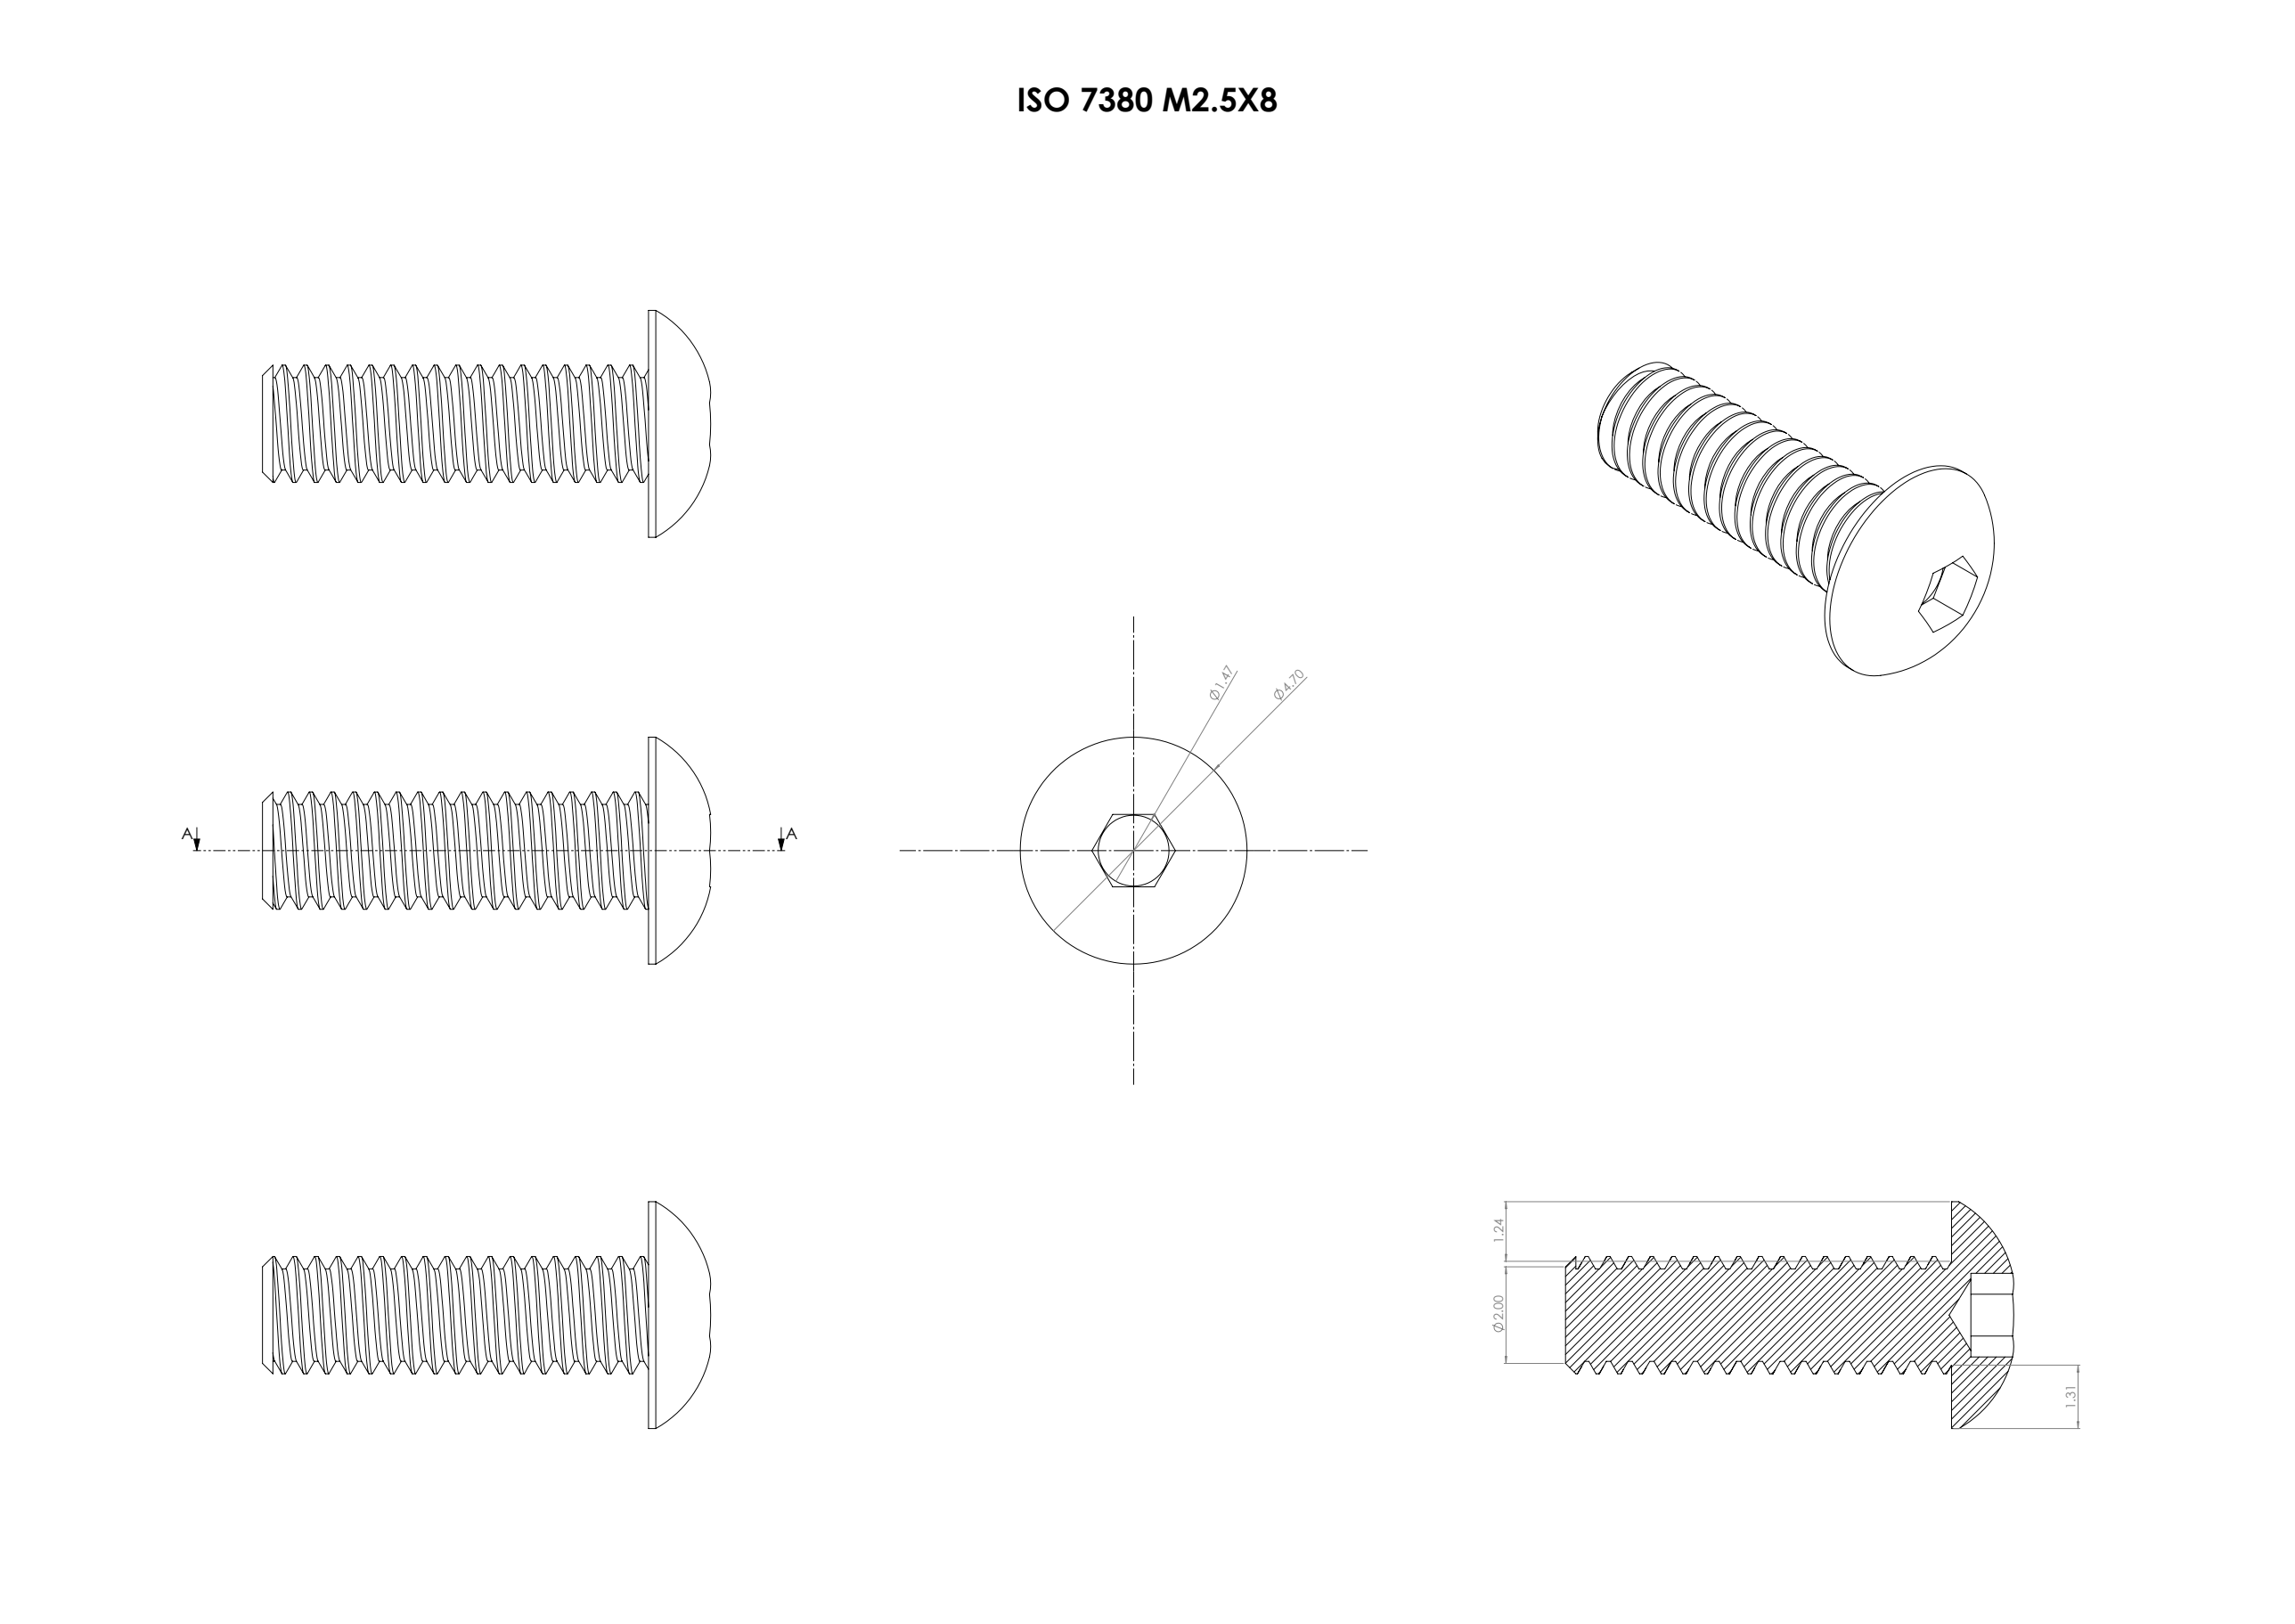
ISO-10303-21;
HEADER;
/* Generated by software containing ST-Developer
 * from STEP Tools, Inc. (www.steptools.com) 
 */

FILE_DESCRIPTION(
/* description */ (''),
/* implementation_level */ '2;1');

FILE_NAME(
/* name */ '13_ISO_7380_M2.5x8.step',
/* time_stamp */ '2026-10-21T02:01:14-07:00',
/* author */ (''),
/* organization */ (''),
/* preprocessor_version */ 'ST-DEVELOPER v20.2',
/* originating_system */ 'Autodesk Translation Framework v15.15.0.0',
/* authorisation */ '');

FILE_SCHEMA (('AUTOMOTIVE_DESIGN { 1 0 10303 214 3 1 1 }'));
ENDSEC;

DATA;
#10=MECHANICAL_DESIGN_GEOMETRIC_PRESENTATION_REPRESENTATION('',(#626),#37181);
#104=(
BOUNDED_SURFACE()
B_SPLINE_SURFACE(2,2,((#37099,#37100,#37101,#37102,#37103,#37104,#37105,
#37106,#37107),(#37108,#37109,#37110,#37111,#37112,#37113,#37114,#37115,
#37116),(#37117,#37118,#37119,#37120,#37121,#37122,#37123,#37124,#37125)),
 .UNSPECIFIED.,.F.,.T.,.F.)
B_SPLINE_SURFACE_WITH_KNOTS((3,3),(3,2,2,2,3),(0.513408172091738,1.39168804086818),
(-3.14159265358979,-1.5707963267949,0.,1.5707963267949,3.14159265358979),
 .UNSPECIFIED.)
GEOMETRIC_REPRESENTATION_ITEM()
RATIONAL_B_SPLINE_SURFACE(((1.,0.707106781186548,1.,0.707106781186548,1.,
0.707106781186548,1.,0.707106781186548,1.),(0.905117664433204,0.640014838292448,
0.905117664433204,0.640014838292448,0.905117664433204,0.640014838292448,
0.905117664433204,0.640014838292448,0.905117664433204),(1.,0.707106781186548,
1.,0.707106781186548,1.,0.707106781186548,1.,0.707106781186548,1.)))
REPRESENTATION_ITEM('')
SURFACE()
);
#118=B_SPLINE_SURFACE_WITH_KNOTS('',3,3,((#35741,#35742,#35743,#35744,#35745,
#35746,#35747,#35748,#35749,#35750,#35751,#35752,#35753,#35754,#35755,#35756,
#35757,#35758,#35759,#35760,#35761,#35762,#35763,#35764,#35765,#35766,#35767,
#35768,#35769,#35770,#35771,#35772,#35773,#35774,#35775,#35776,#35777,#35778,
#35779,#35780,#35781,#35782,#35783,#35784,#35785,#35786,#35787,#35788,#35789,
#35790,#35791,#35792,#35793,#35794,#35795,#35796,#35797,#35798,#35799,#35800,
#35801,#35802,#35803,#35804,#35805,#35806,#35807,#35808,#35809,#35810,#35811,
#35812,#35813,#35814,#35815,#35816,#35817,#35818,#35819,#35820,#35821,#35822,
#35823,#35824,#35825,#35826,#35827,#35828,#35829,#35830,#35831,#35832,#35833,
#35834,#35835,#35836,#35837,#35838,#35839,#35840,#35841,#35842,#35843,#35844,
#35845,#35846,#35847,#35848,#35849,#35850,#35851,#35852,#35853,#35854),
(#35855,#35856,#35857,#35858,#35859,#35860,#35861,#35862,#35863,#35864,
#35865,#35866,#35867,#35868,#35869,#35870,#35871,#35872,#35873,#35874,#35875,
#35876,#35877,#35878,#35879,#35880,#35881,#35882,#35883,#35884,#35885,#35886,
#35887,#35888,#35889,#35890,#35891,#35892,#35893,#35894,#35895,#35896,#35897,
#35898,#35899,#35900,#35901,#35902,#35903,#35904,#35905,#35906,#35907,#35908,
#35909,#35910,#35911,#35912,#35913,#35914,#35915,#35916,#35917,#35918,#35919,
#35920,#35921,#35922,#35923,#35924,#35925,#35926,#35927,#35928,#35929,#35930,
#35931,#35932,#35933,#35934,#35935,#35936,#35937,#35938,#35939,#35940,#35941,
#35942,#35943,#35944,#35945,#35946,#35947,#35948,#35949,#35950,#35951,#35952,
#35953,#35954,#35955,#35956,#35957,#35958,#35959,#35960,#35961,#35962,#35963,
#35964,#35965,#35966,#35967,#35968),(#35969,#35970,#35971,#35972,#35973,
#35974,#35975,#35976,#35977,#35978,#35979,#35980,#35981,#35982,#35983,#35984,
#35985,#35986,#35987,#35988,#35989,#35990,#35991,#35992,#35993,#35994,#35995,
#35996,#35997,#35998,#35999,#36000,#36001,#36002,#36003,#36004,#36005,#36006,
#36007,#36008,#36009,#36010,#36011,#36012,#36013,#36014,#36015,#36016,#36017,
#36018,#36019,#36020,#36021,#36022,#36023,#36024,#36025,#36026,#36027,#36028,
#36029,#36030,#36031,#36032,#36033,#36034,#36035,#36036,#36037,#36038,#36039,
#36040,#36041,#36042,#36043,#36044,#36045,#36046,#36047,#36048,#36049,#36050,
#36051,#36052,#36053,#36054,#36055,#36056,#36057,#36058,#36059,#36060,#36061,
#36062,#36063,#36064,#36065,#36066,#36067,#36068,#36069,#36070,#36071,#36072,
#36073,#36074,#36075,#36076,#36077,#36078,#36079,#36080,#36081,#36082),
(#36083,#36084,#36085,#36086,#36087,#36088,#36089,#36090,#36091,#36092,
#36093,#36094,#36095,#36096,#36097,#36098,#36099,#36100,#36101,#36102,#36103,
#36104,#36105,#36106,#36107,#36108,#36109,#36110,#36111,#36112,#36113,#36114,
#36115,#36116,#36117,#36118,#36119,#36120,#36121,#36122,#36123,#36124,#36125,
#36126,#36127,#36128,#36129,#36130,#36131,#36132,#36133,#36134,#36135,#36136,
#36137,#36138,#36139,#36140,#36141,#36142,#36143,#36144,#36145,#36146,#36147,
#36148,#36149,#36150,#36151,#36152,#36153,#36154,#36155,#36156,#36157,#36158,
#36159,#36160,#36161,#36162,#36163,#36164,#36165,#36166,#36167,#36168,#36169,
#36170,#36171,#36172,#36173,#36174,#36175,#36176,#36177,#36178,#36179,#36180,
#36181,#36182,#36183,#36184,#36185,#36186,#36187,#36188,#36189,#36190,#36191,
#36192,#36193,#36194,#36195,#36196)),.UNSPECIFIED.,.F.,.F.,.F.,(4,4),(4,
1,1,1,1,1,1,1,1,1,1,1,1,1,1,1,1,1,1,1,1,1,1,1,1,1,1,1,1,1,1,1,1,1,1,1,1,
1,1,1,1,1,1,1,1,1,1,1,1,1,1,1,1,1,1,1,1,1,1,1,1,1,1,1,1,1,1,1,1,1,1,1,1,
1,1,1,1,1,1,1,1,1,1,1,1,1,1,1,1,1,1,1,1,1,1,1,1,1,1,1,1,1,1,1,1,1,1,1,1,
1,1,4),(0.,0.0296469363228873),(8.30626835282484,9.30418594221277,10.3021035316007,
11.3000211209886,12.2979387103766,13.2958562997645,14.2937738891524,15.2916914785404,
16.2896090679283,17.2875266573163,18.2854442467042,19.2833618360921,20.2812794254801,
21.279197014868,22.2771146042559,23.2750321936439,24.2729497830318,25.2708673724197,
26.2687849618077,27.2667025511956,28.2646201405835,29.2625377299715,30.2604553193594,
31.2583729087473,32.2562904981353,33.2542080875232,34.2521256769111,35.2500432662991,
36.247960855687,37.245878445075,38.2437960344629,39.2417136238508,40.2396312132388,
41.2375488026267,42.2354663920146,43.2333839814026,44.2313015707905,45.2292191601784,
46.2271367495664,47.2250543389543,48.2229719283422,49.2208895177302,50.2188071071181,
51.216724696506,52.214642285894,53.2125598752819,54.2104774646699,55.2083950540578,
56.2063126434457,57.2042302328337,58.2021478222216,59.2000654116095,60.1979830009975,
61.1959005903854,62.1938181797733,63.1917357691613,64.1896533585492,65.1875709479371,
66.1854885373251,67.183406126713,68.1813237161009,69.1792413054889,70.1771588948768,
71.1750764842647,72.1729940736527,73.1709116630406,74.1688292524286,75.1667468418165,
76.1646644312044,77.1625820205924,78.1604996099803,79.1584171993682,80.1563347887562,
81.1542523781441,82.152169967532,83.15008755692,84.1480051463079,85.1459227356958,
86.1438403250838,87.1417579144717,88.1396755038596,89.1375930932476,90.1355106826355,
91.1334282720235,92.1313458614114,93.1292634507993,94.1271810401873,95.1250986295752,
96.1230162189631,97.1209338083511,98.118851397739,99.1167689871269,100.114686576515,
101.112604165903,102.110521755291,103.108439344679,104.106356934067,105.104274523455,
106.102192112842,107.10010970223,108.098027291618,109.095944881006,110.093862470394,
111.091780059782,112.08969764917,113.087615238558,114.085532827946,115.083450417334,
116.081368006722,117.07928559611,118.077203185498,119.075120774886),
 .UNSPECIFIED.);
#119=B_SPLINE_SURFACE_WITH_KNOTS('',3,3,((#36473,#36474,#36475,#36476,#36477,
#36478,#36479,#36480,#36481,#36482,#36483,#36484,#36485,#36486,#36487,#36488,
#36489,#36490,#36491,#36492,#36493,#36494,#36495,#36496,#36497,#36498,#36499,
#36500,#36501,#36502,#36503,#36504,#36505,#36506,#36507,#36508,#36509,#36510,
#36511,#36512,#36513,#36514,#36515,#36516,#36517,#36518,#36519,#36520,#36521,
#36522,#36523,#36524,#36525,#36526,#36527,#36528,#36529,#36530,#36531,#36532,
#36533,#36534,#36535,#36536,#36537,#36538,#36539,#36540,#36541,#36542,#36543,
#36544,#36545,#36546,#36547,#36548,#36549,#36550,#36551,#36552,#36553,#36554,
#36555,#36556,#36557,#36558,#36559,#36560,#36561,#36562,#36563,#36564,#36565,
#36566,#36567,#36568,#36569,#36570,#36571,#36572,#36573,#36574,#36575,#36576,
#36577,#36578,#36579,#36580,#36581,#36582,#36583,#36584,#36585,#36586),
(#36587,#36588,#36589,#36590,#36591,#36592,#36593,#36594,#36595,#36596,
#36597,#36598,#36599,#36600,#36601,#36602,#36603,#36604,#36605,#36606,#36607,
#36608,#36609,#36610,#36611,#36612,#36613,#36614,#36615,#36616,#36617,#36618,
#36619,#36620,#36621,#36622,#36623,#36624,#36625,#36626,#36627,#36628,#36629,
#36630,#36631,#36632,#36633,#36634,#36635,#36636,#36637,#36638,#36639,#36640,
#36641,#36642,#36643,#36644,#36645,#36646,#36647,#36648,#36649,#36650,#36651,
#36652,#36653,#36654,#36655,#36656,#36657,#36658,#36659,#36660,#36661,#36662,
#36663,#36664,#36665,#36666,#36667,#36668,#36669,#36670,#36671,#36672,#36673,
#36674,#36675,#36676,#36677,#36678,#36679,#36680,#36681,#36682,#36683,#36684,
#36685,#36686,#36687,#36688,#36689,#36690,#36691,#36692,#36693,#36694,#36695,
#36696,#36697,#36698,#36699,#36700),(#36701,#36702,#36703,#36704,#36705,
#36706,#36707,#36708,#36709,#36710,#36711,#36712,#36713,#36714,#36715,#36716,
#36717,#36718,#36719,#36720,#36721,#36722,#36723,#36724,#36725,#36726,#36727,
#36728,#36729,#36730,#36731,#36732,#36733,#36734,#36735,#36736,#36737,#36738,
#36739,#36740,#36741,#36742,#36743,#36744,#36745,#36746,#36747,#36748,#36749,
#36750,#36751,#36752,#36753,#36754,#36755,#36756,#36757,#36758,#36759,#36760,
#36761,#36762,#36763,#36764,#36765,#36766,#36767,#36768,#36769,#36770,#36771,
#36772,#36773,#36774,#36775,#36776,#36777,#36778,#36779,#36780,#36781,#36782,
#36783,#36784,#36785,#36786,#36787,#36788,#36789,#36790,#36791,#36792,#36793,
#36794,#36795,#36796,#36797,#36798,#36799,#36800,#36801,#36802,#36803,#36804,
#36805,#36806,#36807,#36808,#36809,#36810,#36811,#36812,#36813,#36814),
(#36815,#36816,#36817,#36818,#36819,#36820,#36821,#36822,#36823,#36824,
#36825,#36826,#36827,#36828,#36829,#36830,#36831,#36832,#36833,#36834,#36835,
#36836,#36837,#36838,#36839,#36840,#36841,#36842,#36843,#36844,#36845,#36846,
#36847,#36848,#36849,#36850,#36851,#36852,#36853,#36854,#36855,#36856,#36857,
#36858,#36859,#36860,#36861,#36862,#36863,#36864,#36865,#36866,#36867,#36868,
#36869,#36870,#36871,#36872,#36873,#36874,#36875,#36876,#36877,#36878,#36879,
#36880,#36881,#36882,#36883,#36884,#36885,#36886,#36887,#36888,#36889,#36890,
#36891,#36892,#36893,#36894,#36895,#36896,#36897,#36898,#36899,#36900,#36901,
#36902,#36903,#36904,#36905,#36906,#36907,#36908,#36909,#36910,#36911,#36912,
#36913,#36914,#36915,#36916,#36917,#36918,#36919,#36920,#36921,#36922,#36923,
#36924,#36925,#36926,#36927,#36928)),.UNSPECIFIED.,.F.,.F.,.F.,(4,4),(4,
1,1,1,1,1,1,1,1,1,1,1,1,1,1,1,1,1,1,1,1,1,1,1,1,1,1,1,1,1,1,1,1,1,1,1,1,
1,1,1,1,1,1,1,1,1,1,1,1,1,1,1,1,1,1,1,1,1,1,1,1,1,1,1,1,1,1,1,1,1,1,1,1,
1,1,1,1,1,1,1,1,1,1,1,1,1,1,1,1,1,1,1,1,1,1,1,1,1,1,1,1,1,1,1,1,1,1,1,1,
1,1,4),(0.,0.0296469363228873),(11.6151336144495,12.6130512038375,13.6109687932254,
14.6088863826133,15.6068039720013,16.6047215613892,17.6026391507771,18.6005567401651,
19.598474329553,20.5963919189409,21.5943095083289,22.5922270977168,23.5901446871048,
24.5880622764927,25.5859798658806,26.5838974552686,27.5818150446565,28.5797326340444,
29.5776502234324,30.5755678128203,31.5734854022082,32.5714029915962,33.5693205809841,
34.567238170372,35.56515575976,36.5630733491479,37.5609909385358,38.5589085279238,
39.5568261173117,40.5547437066997,41.5526612960876,42.5505788854755,43.5484964748635,
44.5464140642514,45.5443316536393,46.5422492430273,47.5401668324152,48.5380844218031,
49.5360020111911,50.533919600579,51.5318371899669,52.5297547793549,53.5276723687428,
54.5255899581308,55.5235075475187,56.5214251369066,57.5193427262946,58.5172603156825,
59.5151779050704,60.5130954944584,61.5110130838463,62.5089306732342,63.5068482626222,
64.5047658520101,65.502683441398,66.500601030786,67.4985186201739,68.4964362095618,
69.4943537989498,70.4922713883377,71.4901889777257,72.4881065671136,73.4860241565015,
74.4839417458895,75.4818593352774,76.4797769246653,77.4776945140533,78.4756121034412,
79.4735296928291,80.4714472822171,81.469364871605,82.4672824609929,83.4652000503809,
84.4631176397688,85.4610352291567,86.4589528185447,87.4568704079326,88.4547879973206,
89.4527055867085,90.4506231760964,91.4485407654844,92.4464583548723,93.4443759442602,
94.4422935336482,95.4402111230361,96.438128712424,97.436046301812,98.4339638911999,
99.4318814805878,100.429799069976,101.427716659364,102.425634248752,103.42355183814,
104.421469427528,105.419387016915,106.417304606303,107.415222195691,108.413139785079,
109.411057374467,110.408974963855,111.406892553243,112.404810142631,113.402727732019,
114.400645321407,115.398562910795,116.396480500183,117.394398089571,118.392315678959,
119.390233268347,120.388150857734,121.386068447122,122.38398603651),
 .UNSPECIFIED.);
#505=B_SPLINE_CURVE_WITH_KNOTS('',3,(#34463,#34464,#34465,#34466,#34467,
#34468,#34469,#34470,#34471,#34472),.UNSPECIFIED.,.F.,.F.,(4,3,3,4),(-4.09282965349934,
-3.99167035755174,-2.99375276816381,-2.06974660785397),.UNSPECIFIED.);
#506=B_SPLINE_CURVE_WITH_KNOTS('',3,(#34475,#34476,#34477,#34478,#34479,
#34480,#34481),.UNSPECIFIED.,.F.,.F.,(4,3,4),(0.,0.997917589387936,1.11850960794432),
 .UNSPECIFIED.);
#507=B_SPLINE_CURVE_WITH_KNOTS('',3,(#34486,#34487,#34488,#34489,#34490,
#34491,#34492,#34493,#34494,#34495,#34496,#34497,#34498,#34499,#34500,#34501,
#34502,#34503,#34504,#34505,#34506,#34507),.UNSPECIFIED.,.F.,.F.,(4,3,3,
3,3,3,3,4),(-10.3760149606789,-9.97917589387935,-8.98125830449142,-7.98334071510348,
-6.98542312571555,-5.98750553632761,-4.98958794693968,-4.09282965349934),
 .UNSPECIFIED.);
#508=B_SPLINE_CURVE_WITH_KNOTS('',3,(#34508,#34509,#34510,#34511,#34512,
#34513,#34514,#34515,#34516,#34517,#34518,#34519,#34520,#34521,#34522,#34523,
#34524,#34525,#34526,#34527,#34528,#34529),.UNSPECIFIED.,.F.,.F.,(4,3,3,
3,3,3,3,4),(1.11850960794432,1.99583517877587,2.99375276816381,3.99167035755174,
4.98958794693968,5.98750553632761,6.98542312571555,7.40169491512391),
 .UNSPECIFIED.);
#509=B_SPLINE_CURVE_WITH_KNOTS('',3,(#34534,#34535,#34536,#34537,#34538,
#34539,#34540,#34541,#34542,#34543,#34544,#34545,#34546,#34547,#34548,#34549,
#34550,#34551,#34552,#34553,#34554,#34555),.UNSPECIFIED.,.F.,.F.,(4,3,3,
3,3,3,3,4),(-16.6592002678585,-15.966681430207,-14.968763840819,-13.9708462514311,
-12.9729286620432,-11.9750110726552,-10.9770934832673,-10.3760149606789),
 .UNSPECIFIED.);
#510=B_SPLINE_CURVE_WITH_KNOTS('',3,(#34556,#34557,#34558,#34559,#34560,
#34561,#34562,#34563,#34564,#34565,#34566,#34567,#34568,#34569,#34570,#34571,
#34572,#34573,#34574,#34575,#34576,#34577),.UNSPECIFIED.,.F.,.F.,(4,3,3,
3,3,3,3,4),(7.40169491512391,7.98334071510348,8.98125830449142,9.97917589387935,
10.9770934832673,11.9750110726552,12.9729286620432,13.6848802223035),
 .UNSPECIFIED.);
#511=B_SPLINE_CURVE_WITH_KNOTS('',3,(#34582,#34583,#34584,#34585,#34586,
#34587,#34588,#34589,#34590,#34591,#34592,#34593,#34594,#34595,#34596,#34597,
#34598,#34599,#34600,#34601,#34602,#34603),.UNSPECIFIED.,.F.,.F.,(4,3,3,
3,3,3,3,4),(-22.9423855750381,-21.9541869665346,-20.9562693771467,-19.9583517877587,
-18.9604341983708,-17.9625166089828,-16.9645990195949,-16.6592002678585),
 .UNSPECIFIED.);
#512=B_SPLINE_CURVE_WITH_KNOTS('',3,(#34604,#34605,#34606,#34607,#34608,
#34609,#34610,#34611,#34612,#34613,#34614,#34615,#34616,#34617,#34618,#34619,
#34620,#34621,#34622,#34623,#34624,#34625,#34626,#34627,#34628),
 .UNSPECIFIED.,.F.,.F.,(4,3,3,3,3,3,3,3,4),(13.6848802223035,13.9708462514311,
14.968763840819,15.966681430207,16.9645990195949,17.9625166089828,18.9604341983708,
19.9583517877587,19.9680655294831),.UNSPECIFIED.);
#513=B_SPLINE_CURVE_WITH_KNOTS('',3,(#34633,#34634,#34635,#34636,#34637,
#34638,#34639,#34640,#34641,#34642,#34643,#34644,#34645,#34646,#34647,#34648,
#34649,#34650,#34651,#34652,#34653,#34654,#34655,#34656,#34657),
 .UNSPECIFIED.,.F.,.F.,(4,3,3,3,3,3,3,3,4),(-29.2255708822177,-28.9396100922501,
-27.9416925028622,-26.9437749134743,-25.9458573240863,-24.9479397346984,
-23.9500221453105,-22.9521045559225,-22.9423855750381),.UNSPECIFIED.);
#514=B_SPLINE_CURVE_WITH_KNOTS('',3,(#34658,#34659,#34660,#34661,#34662,
#34663,#34664,#34665,#34666,#34667,#34668,#34669,#34670,#34671,#34672,#34673,
#34674,#34675,#34676,#34677,#34678,#34679),.UNSPECIFIED.,.F.,.F.,(4,3,3,
3,3,3,3,4),(19.9680655294831,20.9562693771466,21.9541869665346,22.9521045559225,
23.9500221453104,24.9479397346984,25.9458573240863,26.2512508366627),
 .UNSPECIFIED.);
#515=B_SPLINE_CURVE_WITH_KNOTS('',3,(#34684,#34685,#34686,#34687,#34688,
#34689,#34690,#34691,#34692,#34693,#34694,#34695,#34696,#34697,#34698,#34699,
#34700,#34701,#34702,#34703,#34704,#34705),.UNSPECIFIED.,.F.,.F.,(4,3,3,
3,3,3,3,4),(-35.5087561893973,-34.9271156285777,-33.9291980391898,-32.9312804498019,
-31.9333628604139,-30.935445271026,-29.9375276816381,-29.2255708822177),
 .UNSPECIFIED.);
#516=B_SPLINE_CURVE_WITH_KNOTS('',3,(#34706,#34707,#34708,#34709,#34710,
#34711,#34712,#34713,#34714,#34715,#34716,#34717,#34718,#34719,#34720,#34721,
#34722,#34723,#34724,#34725,#34726,#34727),.UNSPECIFIED.,.F.,.F.,(4,3,3,
3,3,3,3,4),(26.2512508366627,26.9437749134742,27.9416925028622,28.9396100922501,
29.937527681638,30.935445271026,31.9333628604139,32.5344361438423),
 .UNSPECIFIED.);
#517=B_SPLINE_CURVE_WITH_KNOTS('',3,(#34732,#34733,#34734,#34735,#34736,
#34737,#34738,#34739,#34740,#34741,#34742,#34743,#34744,#34745,#34746,#34747,
#34748,#34749,#34750,#34751,#34752,#34753),.UNSPECIFIED.,.F.,.F.,(4,3,3,
3,3,3,3,4),(-41.7919414965769,-40.9146211649053,-39.9167035755174,-38.9187859861295,
-37.9208683967415,-36.9229508073536,-35.9250332179657,-35.5087561893973),
 .UNSPECIFIED.);
#518=B_SPLINE_CURVE_WITH_KNOTS('',3,(#34754,#34755,#34756,#34757,#34758,
#34759,#34760,#34761,#34762,#34763,#34764,#34765,#34766,#34767,#34768,#34769,
#34770,#34771,#34772,#34773,#34774,#34775),.UNSPECIFIED.,.F.,.F.,(4,3,3,
3,3,3,3,4),(32.5344361438423,32.9312804498019,33.9291980391898,34.9271156285777,
35.9250332179657,36.9229508073536,37.9208683967415,38.8176214510219),
 .UNSPECIFIED.);
#519=B_SPLINE_CURVE_WITH_KNOTS('',3,(#34780,#34781,#34782,#34783,#34784,
#34785,#34786,#34787,#34788,#34789,#34790,#34791,#34792,#34793,#34794,#34795,
#34796,#34797,#34798,#34799,#34800,#34801,#34802,#34803,#34804),
 .UNSPECIFIED.,.F.,.F.,(4,3,3,3,3,3,3,3,4),(-48.0751268037565,-47.9000442906209,
-46.902126701233,-45.904209111845,-44.9062915224571,-43.9083739330692,-42.9104563436812,
-41.9125387542933,-41.7919414965769),.UNSPECIFIED.);
#520=B_SPLINE_CURVE_WITH_KNOTS('',3,(#34805,#34806,#34807,#34808,#34809,
#34810,#34811,#34812,#34813,#34814,#34815,#34816,#34817,#34818,#34819,#34820,
#34821,#34822,#34823,#34824,#34825,#34826,#34827,#34828,#34829),
 .UNSPECIFIED.,.F.,.F.,(4,3,3,3,3,3,3,3,4),(38.8176214510219,38.9187859861295,
39.9167035755174,40.9146211649053,41.9125387542933,42.9104563436812,43.9083739330692,
44.9062915224571,45.1008067582014),.UNSPECIFIED.);
#521=B_SPLINE_CURVE_WITH_KNOTS('',3,(#34834,#34835,#34836,#34837,#34838,
#34839,#34840,#34841,#34842,#34843,#34844,#34845,#34846,#34847,#34848,#34849,
#34850,#34851,#34852,#34853,#34854,#34855),.UNSPECIFIED.,.F.,.F.,(4,3,3,
3,3,3,3,4),(-54.358312110936,-53.8875498269485,-52.8896322375606,-51.8917146481726,
-50.8937970587847,-49.8958794693968,-48.8979618800088,-48.0751268037565),
 .UNSPECIFIED.);
#522=B_SPLINE_CURVE_WITH_KNOTS('',3,(#34856,#34857,#34858,#34859,#34860,
#34861,#34862,#34863,#34864,#34865,#34866,#34867,#34868,#34869,#34870,#34871,
#34872,#34873,#34874,#34875,#34876,#34877),.UNSPECIFIED.,.F.,.F.,(4,3,3,
3,3,3,3,4),(45.1008067582014,45.904209111845,46.902126701233,47.9000442906209,
48.8979618800088,49.8958794693968,50.8937970587847,51.383992065381),
 .UNSPECIFIED.);
#523=B_SPLINE_CURVE_WITH_KNOTS('',3,(#34882,#34883,#34884,#34885,#34886,
#34887,#34888,#34889,#34890,#34891,#34892,#34893,#34894,#34895,#34896,#34897,
#34898,#34899,#34900,#34901,#34902,#34903),.UNSPECIFIED.,.F.,.F.,(4,3,3,
3,3,3,3,4),(-60.6414974181156,-59.8750553632761,-58.8771377738882,-57.8792201845003,
-56.8813025951123,-55.8833850057244,-54.8854674163365,-54.358312110936),
 .UNSPECIFIED.);
#524=B_SPLINE_CURVE_WITH_KNOTS('',3,(#34904,#34905,#34906,#34907,#34908,
#34909,#34910,#34911,#34912,#34913,#34914,#34915,#34916,#34917,#34918,#34919,
#34920,#34921,#34922,#34923,#34924,#34925),.UNSPECIFIED.,.F.,.F.,(4,3,3,
3,3,3,3,4),(51.383992065381,51.8917146481726,52.8896322375606,53.8875498269485,
54.8854674163364,55.8833850057244,56.8813025951123,57.6671773725606),
 .UNSPECIFIED.);
#525=B_SPLINE_CURVE_WITH_KNOTS('',3,(#34930,#34931,#34932,#34933,#34934,
#34935,#34936,#34937,#34938,#34939,#34940,#34941,#34942,#34943,#34944,#34945,
#34946,#34947,#34948,#34949,#34950,#34951,#34952,#34953,#34954),
 .UNSPECIFIED.,.F.,.F.,(4,3,3,3,3,3,3,3,4),(-66.9246827252952,-66.8604784889917,
-65.8625608996037,-64.8646433102158,-63.8667257208279,-62.8688081314399,
-61.870890542052,-60.8729729526641,-60.6414974181156),.UNSPECIFIED.);
#526=B_SPLINE_CURVE_WITH_KNOTS('',3,(#34955,#34956,#34957,#34958,#34959,
#34960,#34961,#34962,#34963,#34964,#34965,#34966,#34967,#34968,#34969,#34970,
#34971,#34972,#34973,#34974,#34975,#34976,#34977,#34978,#34979),
 .UNSPECIFIED.,.F.,.F.,(4,3,3,3,3,3,3,3,4),(57.6671773725606,57.8792201845002,
58.8771377738882,59.8750553632761,60.872972952664,61.870890542052,62.8688081314399,
63.8667257208279,63.9503626797402),.UNSPECIFIED.);
#527=B_SPLINE_CURVE_WITH_KNOTS('',3,(#34984,#34985,#34986,#34987,#34988,
#34989,#34990,#34991,#34992,#34993,#34994,#34995,#34996,#34997,#34998,#34999,
#35000,#35001,#35002,#35003,#35004,#35005),.UNSPECIFIED.,.F.,.F.,(4,3,3,
3,3,3,3,4),(-73.2078680324748,-72.8479840253193,-71.8500664359313,-70.8521488465434,
-69.8542312571555,-68.8563136677676,-67.8583960783796,-66.9246827252952),
 .UNSPECIFIED.);
#528=B_SPLINE_CURVE_WITH_KNOTS('',3,(#35006,#35007,#35008,#35009,#35010,
#35011,#35012,#35013,#35014,#35015,#35016,#35017,#35018,#35019,#35020,#35021,
#35022,#35023,#35024,#35025,#35026,#35027),.UNSPECIFIED.,.F.,.F.,(4,3,3,
3,3,3,3,4),(63.9503626797402,64.8646433102158,65.8625608996037,66.8604784889917,
67.8583960783796,68.8563136677676,69.8542312571555,70.2335479869198),
 .UNSPECIFIED.);
#529=B_SPLINE_CURVE_WITH_KNOTS('',3,(#35032,#35033,#35034,#35035,#35036,
#35037,#35038,#35039,#35040,#35041,#35042,#35043,#35044,#35045,#35046,#35047,
#35048,#35049,#35050,#35051,#35052,#35053),.UNSPECIFIED.,.F.,.F.,(4,3,3,
3,3,3,3,4),(-79.4910533396544,-78.8354895616469,-77.837571972259,-76.839654382871,
-75.8417367934831,-74.8438192040951,-73.8459016147072,-73.2078680324748),
 .UNSPECIFIED.);
#530=B_SPLINE_CURVE_WITH_KNOTS('',3,(#35054,#35055,#35056,#35057,#35058,
#35059,#35060,#35061,#35062,#35063,#35064,#35065,#35066,#35067,#35068,#35069,
#35070,#35071,#35072,#35073,#35074,#35075),.UNSPECIFIED.,.F.,.F.,(4,3,3,
3,3,3,3,4),(70.2335479869198,70.8521488465434,71.8500664359314,72.8479840253193,
73.8459016147072,74.8438192040951,75.8417367934831,76.5167332940994),
 .UNSPECIFIED.);
#531=B_SPLINE_CURVE_WITH_KNOTS('',3,(#35080,#35081,#35082,#35083,#35084,
#35085,#35086,#35087,#35088,#35089,#35090,#35091,#35092,#35093,#35094,#35095,
#35096,#35097,#35098,#35099,#35100,#35101),.UNSPECIFIED.,.F.,.F.,(4,3,3,
3,3,3,3,4),(-85.774238646834,-84.8229950979745,-83.8250775085866,-82.8271599191986,
-81.8292423298107,-80.8313247404228,-79.8334071510348,-79.4910533396544),
 .UNSPECIFIED.);
#532=B_SPLINE_CURVE_WITH_KNOTS('',3,(#35102,#35103,#35104,#35105,#35106,
#35107,#35108,#35109,#35110,#35111,#35112,#35113,#35114,#35115,#35116,#35117,
#35118,#35119,#35120,#35121,#35122,#35123),.UNSPECIFIED.,.F.,.F.,(4,3,3,
3,3,3,3,4),(76.5167332940994,76.839654382871,77.8375719722589,78.8354895616469,
79.8334071510348,80.8313247404228,81.8292423298107,82.799918601279),
 .UNSPECIFIED.);
#533=B_SPLINE_CURVE_WITH_KNOTS('',3,(#35128,#35129,#35130,#35131,#35132,
#35133,#35134,#35135,#35136,#35137,#35138,#35139,#35140,#35141,#35142,#35143,
#35144,#35145,#35146,#35147,#35148,#35149,#35150,#35151,#35152),
 .UNSPECIFIED.,.F.,.F.,(4,3,3,3,3,3,3,3,4),(-92.0574239540136,-91.8084182236901,
-90.8105006343021,-89.8125830449142,-88.8146654555263,-87.8167478661383,
-86.8188302767504,-85.8209126873625,-85.774238646834),.UNSPECIFIED.);
#534=B_SPLINE_CURVE_WITH_KNOTS('',3,(#35153,#35154,#35155,#35156,#35157,
#35158,#35159,#35160,#35161,#35162,#35163,#35164,#35165,#35166,#35167,#35168,
#35169,#35170,#35171,#35172,#35173,#35174,#35175,#35176,#35177),
 .UNSPECIFIED.,.F.,.F.,(4,3,3,3,3,3,3,3,4),(82.799918601279,82.8271599191986,
83.8250775085866,84.8229950979745,85.8209126873624,86.8188302767503,87.8167478661383,
88.8146654555262,89.0831039084586),.UNSPECIFIED.);
#535=B_SPLINE_CURVE_WITH_KNOTS('',3,(#35182,#35183,#35184,#35185,#35186,
#35187,#35188,#35189,#35190,#35191,#35192,#35193,#35194,#35195,#35196,#35197,
#35198,#35199,#35200,#35201,#35202,#35203),.UNSPECIFIED.,.F.,.F.,(4,3,3,
3,3,3,3,4),(-98.3406092611932,-97.7959237600177,-96.7980061706297,-95.8000885812418,
-94.8021709918539,-93.8042534024659,-92.806335813078,-92.0574239540136),
 .UNSPECIFIED.);
#536=B_SPLINE_CURVE_WITH_KNOTS('',3,(#35204,#35205,#35206,#35207,#35208,
#35209,#35210,#35211,#35212,#35213,#35214,#35215,#35216,#35217,#35218,#35219,
#35220,#35221,#35222,#35223,#35224,#35225),.UNSPECIFIED.,.F.,.F.,(4,3,3,
3,3,3,3,4),(89.0831039084586,89.8125830449142,90.8105006343021,91.80841822369,
92.806335813078,93.8042534024659,94.8021709918538,95.3662892156382),
 .UNSPECIFIED.);
#537=B_SPLINE_CURVE_WITH_KNOTS('',3,(#35230,#35231,#35232,#35233,#35234,
#35235,#35236,#35237,#35238,#35239,#35240,#35241,#35242,#35243,#35244,#35245,
#35246,#35247,#35248,#35249,#35250,#35251),.UNSPECIFIED.,.F.,.F.,(4,3,3,
3,3,3,3,4),(-104.623794568373,-103.783429296345,-102.785511706957,-101.787594117569,
-100.789676528181,-99.7917589387935,-98.7938413494056,-98.3406092611932),
 .UNSPECIFIED.);
#538=B_SPLINE_CURVE_WITH_KNOTS('',3,(#35252,#35253,#35254,#35255,#35256,
#35257,#35258,#35259,#35260,#35261,#35262,#35263,#35264,#35265,#35266,#35267,
#35268,#35269,#35270,#35271,#35272,#35273),.UNSPECIFIED.,.F.,.F.,(4,3,3,
3,3,3,3,4),(95.3662892156382,95.8000885812418,96.7980061706297,97.7959237600176,
98.7938413494056,99.7917589387935,100.789676528181,101.649474522818),
 .UNSPECIFIED.);
#539=B_SPLINE_CURVE_WITH_KNOTS('',3,(#35280,#35281,#35282,#35283,#35284,
#35285,#35286,#35287,#35288,#35289,#35290,#35291,#35292,#35293,#35294,#35295,
#35296,#35297,#35298,#35299,#35300,#35301),.UNSPECIFIED.,.F.,.F.,(4,3,3,
3,3,3,3,4),(-110.768852422061,-109.770934832673,-108.773017243285,-107.775099653897,
-106.777182064509,-105.779264475121,-104.781346885733,-104.623794568373),
 .UNSPECIFIED.);
#540=B_SPLINE_CURVE_WITH_KNOTS('',3,(#35302,#35303,#35304,#35305,#35306,
#35307,#35308,#35309,#35310,#35311,#35312,#35313,#35314,#35315,#35316,#35317,
#35318,#35319,#35320,#35321,#35322,#35323,#35324,#35325,#35326),
 .UNSPECIFIED.,.F.,.F.,(4,3,3,3,3,3,3,3,4),(101.649474522818,101.787594117569,
102.785511706957,103.783429296345,104.781346885733,105.779264475121,106.777182064509,
107.775099653897,107.932659829997),.UNSPECIFIED.);
#541=B_SPLINE_CURVE_WITH_KNOTS('',3,(#35332,#35333,#35334,#35335,#35336,
#35337,#35338,#35339),.UNSPECIFIED.,.F.,.F.,(4,1,1,1,1,4),(116.238928182822,
116.396480500183,117.394398089571,118.392315678959,119.390233268347,120.314239428656),
 .UNSPECIFIED.);
#542=B_SPLINE_CURVE_WITH_KNOTS('',3,(#35342,#35343,#35344,#35345,#35346,
#35347),.UNSPECIFIED.,.F.,.F.,(4,1,1,4),(116.238928182822,117.07928559611,
118.077203185498,119.075120774886),.UNSPECIFIED.);
#543=B_SPLINE_CURVE_WITH_KNOTS('',3,(#35352,#35353,#35354,#35355,#35356,
#35357,#35358,#35359,#35360,#35361),.UNSPECIFIED.,.F.,.F.,(4,1,1,1,1,1,
1,4),(109.955742875643,110.408974963855,111.406892553243,112.404810142631,
113.402727732019,114.400645321407,115.398562910795,116.238928182822),
 .UNSPECIFIED.);
#544=B_SPLINE_CURVE_WITH_KNOTS('',3,(#35362,#35363,#35364,#35365,#35366,
#35367,#35368,#35369,#35370,#35371,#35372),.UNSPECIFIED.,.F.,.F.,(4,1,1,
1,1,1,1,1,4),(109.955742875643,110.093862470394,111.091780059782,112.08969764917,
113.087615238558,114.085532827946,115.083450417334,116.081368006722,116.238928182822),
 .UNSPECIFIED.);
#545=B_SPLINE_CURVE_WITH_KNOTS('',3,(#35377,#35378,#35379,#35380,#35381,
#35382,#35383,#35384,#35385,#35386),.UNSPECIFIED.,.F.,.F.,(4,1,1,1,1,1,
1,4),(103.672557568463,104.421469427528,105.419387016915,106.417304606303,
107.415222195691,108.413139785079,109.411057374467,109.955742875643),
 .UNSPECIFIED.);
#546=B_SPLINE_CURVE_WITH_KNOTS('',3,(#35387,#35388,#35389,#35390,#35391,
#35392,#35393,#35394,#35395,#35396),.UNSPECIFIED.,.F.,.F.,(4,1,1,1,1,1,
1,4),(103.672557568463,104.106356934067,105.104274523455,106.102192112842,
107.10010970223,108.098027291618,109.095944881006,109.955742875643),
 .UNSPECIFIED.);
#547=B_SPLINE_CURVE_WITH_KNOTS('',3,(#35401,#35402,#35403,#35404,#35405,
#35406,#35407,#35408,#35409,#35410,#35411),.UNSPECIFIED.,.F.,.F.,(4,1,1,
1,1,1,1,1,4),(97.3893722612836,97.436046301812,98.4339638911999,99.4318814805878,
100.429799069976,101.427716659364,102.425634248752,103.42355183814,103.672557568463),
 .UNSPECIFIED.);
#548=B_SPLINE_CURVE_WITH_KNOTS('',3,(#35412,#35413,#35414,#35415,#35416,
#35417,#35418,#35419,#35420,#35421),.UNSPECIFIED.,.F.,.F.,(4,1,1,1,1,1,
1,4),(97.3893722612836,98.118851397739,99.1167689871269,100.114686576515,
101.112604165903,102.110521755291,103.108439344679,103.672557568463),
 .UNSPECIFIED.);
#549=B_SPLINE_CURVE_WITH_KNOTS('',3,(#35426,#35427,#35428,#35429,#35430,
#35431,#35432,#35433,#35434,#35435),.UNSPECIFIED.,.F.,.F.,(4,1,1,1,1,1,
1,4),(91.106186954104,91.4485407654844,92.4464583548723,93.4443759442602,
94.4422935336482,95.4402111230361,96.438128712424,97.3893722612836),
 .UNSPECIFIED.);
#550=B_SPLINE_CURVE_WITH_KNOTS('',3,(#35436,#35437,#35438,#35439,#35440,
#35441,#35442,#35443,#35444,#35445,#35446),.UNSPECIFIED.,.F.,.F.,(4,1,1,
1,1,1,1,1,4),(91.106186954104,91.1334282720235,92.1313458614114,93.1292634507993,
94.1271810401873,95.1250986295752,96.1230162189631,97.1209338083511,97.3893722612836),
 .UNSPECIFIED.);
#551=B_SPLINE_CURVE_WITH_KNOTS('',3,(#35451,#35452,#35453,#35454,#35455,
#35456,#35457,#35458,#35459,#35460),.UNSPECIFIED.,.F.,.F.,(4,1,1,1,1,1,
1,4),(84.8230016469244,85.4610352291567,86.4589528185447,87.4568704079326,
88.4547879973206,89.4527055867085,90.4506231760964,91.106186954104),
 .UNSPECIFIED.);
#552=B_SPLINE_CURVE_WITH_KNOTS('',3,(#35461,#35462,#35463,#35464,#35465,
#35466,#35467,#35468,#35469,#35470),.UNSPECIFIED.,.F.,.F.,(4,1,1,1,1,1,
1,4),(84.8230016469244,85.1459227356958,86.1438403250838,87.1417579144717,
88.1396755038596,89.1375930932476,90.1355106826355,91.106186954104),
 .UNSPECIFIED.);
#553=B_SPLINE_CURVE_WITH_KNOTS('',3,(#35475,#35476,#35477,#35478,#35479,
#35480,#35481,#35482,#35483,#35484),.UNSPECIFIED.,.F.,.F.,(4,1,1,1,1,1,
1,4),(78.5398163397448,79.4735296928291,80.4714472822171,81.469364871605,
82.4672824609929,83.4652000503809,84.4631176397688,84.8230016469244),
 .UNSPECIFIED.);
#554=B_SPLINE_CURVE_WITH_KNOTS('',3,(#35485,#35486,#35487,#35488,#35489,
#35490,#35491,#35492,#35493,#35494),.UNSPECIFIED.,.F.,.F.,(4,1,1,1,1,1,
1,4),(78.5398163397448,79.1584171993682,80.1563347887562,81.1542523781441,
82.152169967532,83.15008755692,84.1480051463079,84.8230016469244),
 .UNSPECIFIED.);
#555=B_SPLINE_CURVE_WITH_KNOTS('',3,(#35499,#35500,#35501,#35502,#35503,
#35504,#35505,#35506,#35507,#35508,#35509),.UNSPECIFIED.,.F.,.F.,(4,1,1,
1,1,1,1,1,4),(72.2566310325652,72.4881065671136,73.4860241565015,74.4839417458895,
75.4818593352774,76.4797769246653,77.4776945140533,78.4756121034412,78.5398163397448),
 .UNSPECIFIED.);
#556=B_SPLINE_CURVE_WITH_KNOTS('',3,(#35510,#35511,#35512,#35513,#35514,
#35515,#35516,#35517,#35518,#35519),.UNSPECIFIED.,.F.,.F.,(4,1,1,1,1,1,
1,4),(72.2566310325652,73.1709116630406,74.1688292524286,75.1667468418165,
76.1646644312044,77.1625820205924,78.1604996099803,78.5398163397448),
 .UNSPECIFIED.);
#557=B_SPLINE_CURVE_WITH_KNOTS('',3,(#35524,#35525,#35526,#35527,#35528,
#35529,#35530,#35531,#35532,#35533),.UNSPECIFIED.,.F.,.F.,(4,1,1,1,1,1,
1,4),(65.9734457253856,66.500601030786,67.4985186201739,68.4964362095618,
69.4943537989498,70.4922713883377,71.4901889777257,72.2566310325652),
 .UNSPECIFIED.);
#558=B_SPLINE_CURVE_WITH_KNOTS('',3,(#35534,#35535,#35536,#35537,#35538,
#35539,#35540,#35541,#35542,#35543,#35544),.UNSPECIFIED.,.F.,.F.,(4,1,1,
1,1,1,1,1,4),(65.9734457253856,66.1854885373251,67.183406126713,68.1813237161009,
69.1792413054889,70.1771588948768,71.1750764842647,72.1729940736527,72.2566310325652),
 .UNSPECIFIED.);
#559=B_SPLINE_CURVE_WITH_KNOTS('',3,(#35549,#35550,#35551,#35552,#35553,
#35554,#35555,#35556,#35557,#35558),.UNSPECIFIED.,.F.,.F.,(4,1,1,1,1,1,
1,4),(59.690260418206,60.5130954944584,61.5110130838463,62.5089306732342,
63.5068482626222,64.5047658520101,65.502683441398,65.9734457253856),
 .UNSPECIFIED.);
#560=B_SPLINE_CURVE_WITH_KNOTS('',3,(#35559,#35560,#35561,#35562,#35563,
#35564,#35565,#35566,#35567,#35568),.UNSPECIFIED.,.F.,.F.,(4,1,1,1,1,1,
1,4),(59.690260418206,60.1979830009975,61.1959005903854,62.1938181797733,
63.1917357691613,64.1896533585492,65.1875709479371,65.9734457253856),
 .UNSPECIFIED.);
#561=B_SPLINE_CURVE_WITH_KNOTS('',3,(#35573,#35574,#35575,#35576,#35577,
#35578,#35579,#35580,#35581,#35582,#35583),.UNSPECIFIED.,.F.,.F.,(4,1,1,
1,1,1,1,1,4),(53.4070751110264,53.5276723687428,54.5255899581308,55.5235075475187,
56.5214251369066,57.5193427262946,58.5172603156825,59.5151779050704,59.690260418206),
 .UNSPECIFIED.);
#562=B_SPLINE_CURVE_WITH_KNOTS('',3,(#35584,#35585,#35586,#35587,#35588,
#35589,#35590,#35591,#35592,#35593),.UNSPECIFIED.,.F.,.F.,(4,1,1,1,1,1,
1,4),(53.4070751110264,54.2104774646699,55.2083950540578,56.2063126434457,
57.2042302328337,58.2021478222216,59.2000654116095,59.690260418206),
 .UNSPECIFIED.);
#563=B_SPLINE_CURVE_WITH_KNOTS('',3,(#35598,#35599,#35600,#35601,#35602,
#35603,#35604,#35605,#35606,#35607),.UNSPECIFIED.,.F.,.F.,(4,1,1,1,1,1,
1,4),(47.1238898038469,47.5401668324152,48.5380844218031,49.5360020111911,
50.533919600579,51.5318371899669,52.5297547793549,53.4070751110264),
 .UNSPECIFIED.);
#564=B_SPLINE_CURVE_WITH_KNOTS('',3,(#35608,#35609,#35610,#35611,#35612,
#35613,#35614,#35615,#35616,#35617,#35618),.UNSPECIFIED.,.F.,.F.,(4,1,1,
1,1,1,1,1,4),(47.1238898038468,47.2250543389543,48.2229719283422,49.2208895177302,
50.2188071071181,51.216724696506,52.214642285894,53.2125598752819,53.4070751110264),
 .UNSPECIFIED.);
#565=B_SPLINE_CURVE_WITH_KNOTS('',3,(#35623,#35624,#35625,#35626,#35627,
#35628,#35629,#35630,#35631,#35632),.UNSPECIFIED.,.F.,.F.,(4,1,1,1,1,1,
1,4),(40.8407044966672,41.5526612960876,42.5505788854755,43.5484964748635,
44.5464140642514,45.5443316536393,46.5422492430273,47.1238898038469),
 .UNSPECIFIED.);
#566=B_SPLINE_CURVE_WITH_KNOTS('',3,(#35633,#35634,#35635,#35636,#35637,
#35638,#35639,#35640,#35641,#35642),.UNSPECIFIED.,.F.,.F.,(4,1,1,1,1,1,
1,4),(40.8407044966672,41.2375488026267,42.2354663920146,43.2333839814026,
44.2313015707905,45.2292191601784,46.2271367495664,47.1238898038468),
 .UNSPECIFIED.);
#567=B_SPLINE_CURVE_WITH_KNOTS('',3,(#35647,#35648,#35649,#35650,#35651,
#35652,#35653,#35654,#35655,#35656,#35657),.UNSPECIFIED.,.F.,.F.,(4,1,1,
1,1,1,1,1,4),(34.5575191894876,34.567238170372,35.56515575976,36.5630733491479,
37.5609909385358,38.5589085279238,39.5568261173117,40.5547437066997,40.8407044966672),
 .UNSPECIFIED.);
#568=B_SPLINE_CURVE_WITH_KNOTS('',3,(#35658,#35659,#35660,#35661,#35662,
#35663,#35664,#35665,#35666,#35667),.UNSPECIFIED.,.F.,.F.,(4,1,1,1,1,1,
1,4),(34.5575191894876,35.2500432662991,36.247960855687,37.245878445075,
38.2437960344629,39.2417136238508,40.2396312132388,40.8407044966672),
 .UNSPECIFIED.);
#569=B_SPLINE_CURVE_WITH_KNOTS('',3,(#35672,#35673,#35674,#35675,#35676,
#35677,#35678,#35679,#35680,#35681),.UNSPECIFIED.,.F.,.F.,(4,1,1,1,1,1,
1,4),(28.2743338823081,28.5797326340444,29.5776502234324,30.5755678128203,
31.5734854022082,32.5714029915962,33.5693205809841,34.5575191894876),
 .UNSPECIFIED.);
#570=B_SPLINE_CURVE_WITH_KNOTS('',3,(#35682,#35683,#35684,#35685,#35686,
#35687,#35688,#35689,#35690,#35691),.UNSPECIFIED.,.F.,.F.,(4,1,1,1,1,1,
1,4),(28.2743338823081,29.2625377299715,30.2604553193594,31.2583729087473,
32.2562904981353,33.2542080875232,34.2521256769111,34.5575191894876),
 .UNSPECIFIED.);
#571=B_SPLINE_CURVE_WITH_KNOTS('',3,(#35696,#35697,#35698,#35699,#35700,
#35701,#35702,#35703,#35704,#35705),.UNSPECIFIED.,.F.,.F.,(4,1,1,1,1,1,
1,4),(21.9911485751285,22.5922270977168,23.5901446871048,24.5880622764927,
25.5859798658806,26.5838974552686,27.5818150446565,28.2743338823081),
 .UNSPECIFIED.);
#572=B_SPLINE_CURVE_WITH_KNOTS('',3,(#35706,#35707,#35708,#35709,#35710,
#35711,#35712,#35713,#35714,#35715,#35716),.UNSPECIFIED.,.F.,.F.,(4,1,1,
1,1,1,1,1,4),(21.9911485751285,22.2771146042559,23.2750321936439,24.2729497830318,
25.2708673724197,26.2687849618077,27.2667025511956,28.2646201405835,28.2743338823081),
 .UNSPECIFIED.);
#573=B_SPLINE_CURVE_WITH_KNOTS('',3,(#35721,#35722,#35723,#35724,#35725,
#35726,#35727,#35728,#35729,#35730),.UNSPECIFIED.,.F.,.F.,(4,1,1,1,1,1,
1,4),(15.7079632679489,16.6047215613892,17.6026391507771,18.6005567401651,
19.598474329553,20.5963919189409,21.5943095083289,21.9911485751285),
 .UNSPECIFIED.);
#574=B_SPLINE_CURVE_WITH_KNOTS('',3,(#35731,#35732,#35733,#35734,#35735,
#35736,#35737,#35738,#35739,#35740),.UNSPECIFIED.,.F.,.F.,(4,1,1,1,1,1,
1,4),(15.7079632679489,16.2896090679283,17.2875266573163,18.2854442467042,
19.2833618360921,20.2812794254801,21.279197014868,21.9911485751285),
 .UNSPECIFIED.);
#575=B_SPLINE_CURVE_WITH_KNOTS('',3,(#36198,#36199,#36200,#36201,#36202,
#36203,#36204,#36205,#36206,#36207,#36208,#36209,#36210,#36211,#36212,#36213,
#36214,#36215,#36216,#36217,#36218,#36219,#36220,#36221,#36222,#36223,#36224,
#36225,#36226,#36227,#36228,#36229,#36230,#36231,#36232,#36233,#36234,#36235,
#36236,#36237,#36238,#36239,#36240,#36241,#36242,#36243,#36244,#36245,#36246,
#36247,#36248,#36249,#36250,#36251,#36252,#36253,#36254,#36255,#36256,#36257,
#36258,#36259,#36260,#36261,#36262,#36263,#36264,#36265,#36266,#36267,#36268,
#36269,#36270,#36271,#36272,#36273,#36274,#36275,#36276,#36277,#36278,#36279),
 .UNSPECIFIED.,.F.,.F.,(4,3,3,3,3,3,3,3,3,3,3,3,3,3,3,3,3,3,3,3,3,3,3,3,
3,3,3,4),(-0.226379821609609,-0.217417340914373,-0.203083213732059,-0.195372161893588,
-0.192039947119467,-0.177142411517304,-0.167842650509623,-0.163493959889746,
-0.160580088349981,-0.14612114712645,-0.132066803420463,-0.124736183429312,
-0.120417462119026,-0.117749049396246,-0.10410960904933,-0.10274432345586,
-0.0897927198647197,-0.0833430124220497,-0.0779132429380391,-0.0753020462900725,
-0.0617532421277136,-0.0483128407128765,-0.0422737356237669,-0.0385418519188507,
-0.0362561171872797,-0.0233422370406623,-0.010890275470702,0.),
 .UNSPECIFIED.);
#576=B_SPLINE_CURVE_WITH_KNOTS('',3,(#36280,#36281,#36282,#36283),
 .UNSPECIFIED.,.F.,.F.,(4,4),(107.932659829997,108.699105814207),
 .UNSPECIFIED.);
#577=B_SPLINE_CURVE_WITH_KNOTS('',3,(#36285,#36286,#36287,#36288,#36289,
#36290,#36291,#36292,#36293,#36294,#36295,#36296,#36297,#36298,#36299,#36300,
#36301,#36302,#36303,#36304,#36305,#36306,#36307,#36308,#36309,#36310,#36311,
#36312,#36313,#36314,#36315,#36316,#36317,#36318,#36319,#36320,#36321,#36322,
#36323,#36324,#36325,#36326,#36327,#36328,#36329,#36330,#36331,#36332,#36333,
#36334,#36335,#36336,#36337,#36338,#36339,#36340,#36341,#36342,#36343,#36344,
#36345,#36346,#36347,#36348,#36349,#36350,#36351,#36352,#36353,#36354,#36355,
#36356,#36357,#36358,#36359,#36360,#36361,#36362,#36363,#36364,#36365,#36366),
 .UNSPECIFIED.,.F.,.F.,(4,3,3,3,3,3,3,3,3,3,3,3,3,3,3,3,3,3,3,3,3,3,3,3,
3,3,3,4),(-0.227523845437319,-0.220310172333792,-0.207301707943979,-0.203017170993446,
-0.199143852533238,-0.186050942785289,-0.177324882089039,-0.174438766917075,
-0.171551170337076,-0.15772399205663,-0.143919217003735,-0.137000027056623,
-0.134028108119541,-0.131666540053468,-0.11740868074808,-0.11624245721529,
-0.102496756909348,-0.0956119105440934,-0.0920583895072349,-0.0888709289525678,
-0.0745568929340286,-0.0599189450724288,-0.0524290769383752,-0.0472022677637861,
-0.0444388522067339,-0.0293009632710678,-0.0142728712478951,0.),
 .UNSPECIFIED.);
#578=B_SPLINE_CURVE_WITH_KNOTS('',3,(#36367,#36368,#36369,#36370,#36371,
#36372,#36373,#36374,#36375),.UNSPECIFIED.,.F.,.F.,(4,1,1,1,1,1,4),(10.3760149606788,
11.3000211209886,12.2979387103766,13.2958562997645,14.2937738891524,15.2916914785404,
15.7079632679489),.UNSPECIFIED.);
#579=B_SPLINE_CURVE_WITH_KNOTS('',3,(#36381,#36382,#36383,#36384,#36385,
#36386,#36387,#36388,#36389,#36390,#36391,#36392,#36393,#36394,#36395,#36396,
#36397,#36398,#36399,#36400,#36401,#36402,#36403,#36404,#36405,#36406,#36407,
#36408,#36409,#36410,#36411,#36412,#36413,#36414,#36415,#36416,#36417,#36418,
#36419,#36420,#36421,#36422,#36423,#36424,#36425,#36426,#36427,#36428,#36429,
#36430,#36431,#36432,#36433,#36434,#36435,#36436,#36437,#36438,#36439,#36440,
#36441,#36442,#36443,#36444,#36445,#36446,#36447,#36448,#36449,#36450,#36451,
#36452,#36453,#36454,#36455,#36456,#36457,#36458,#36459,#36460,#36461,#36462),
 .UNSPECIFIED.,.F.,.F.,(4,3,3,3,3,3,3,3,3,3,3,3,3,3,3,3,3,3,3,3,3,3,3,3,
3,3,3,4),(-0.226379821609595,-0.217417340914356,-0.203083213732043,-0.195372160903899,
-0.192039946137513,-0.17714241040132,-0.167842649533136,-0.163493952881452,
-0.16058007692827,-0.146121138560165,-0.132066791448452,-0.124736174450301,
-0.12041746383325,-0.117749050048006,-0.10410960636557,-0.10274432345585,
-0.089792743953128,-0.0833430503489106,-0.0779136525561493,-0.0753021579254146,
-0.0617533538087251,-0.048312953095273,-0.0422738339583639,-0.0385420785344113,
-0.0362564590884195,-0.023342576751842,-0.0108906149115675,0.),
 .UNSPECIFIED.);
#580=B_SPLINE_CURVE_WITH_KNOTS('',3,(#36465,#36466,#36467,#36468,#36469,
#36470,#36471,#36472),.UNSPECIFIED.,.F.,.F.,(4,1,1,1,1,4),(11.6151336144495,
12.6130512038375,13.6109687932254,14.6088863826133,15.6068039720013,15.7079632679489),
 .UNSPECIFIED.);
#581=B_SPLINE_CURVE_WITH_KNOTS('',3,(#36929,#36930,#36931,#36932,#36933,
#36934,#36935,#36936,#36937,#36938,#36939,#36940,#36941,#36942,#36943,#36944,
#36945,#36946,#36947,#36948,#36949,#36950,#36951,#36952,#36953,#36954,#36955,
#36956,#36957,#36958,#36959,#36960,#36961,#36962,#36963,#36964,#36965,#36966,
#36967,#36968,#36969,#36970,#36971,#36972,#36973,#36974,#36975,#36976,#36977,
#36978,#36979,#36980,#36981,#36982,#36983,#36984,#36985,#36986,#36987,#36988,
#36989,#36990,#36991,#36992,#36993,#36994,#36995,#36996,#36997,#36998,#36999,
#37000,#37001,#37002,#37003,#37004,#37005,#37006,#37007,#37008,#37009,#37010),
 .UNSPECIFIED.,.F.,.F.,(4,3,3,3,3,3,3,3,3,3,3,3,3,3,3,3,3,3,3,3,3,3,3,3,
3,3,3,4),(-0.227523845437348,-0.220310172333817,-0.207301707944002,-0.203017167295075,
-0.199143851355958,-0.186050939006339,-0.177324878782459,-0.174438745964263,
-0.171551166758963,-0.157723989373046,-0.143919214553493,-0.137000025218943,
-0.134028090264727,-0.131666515493408,-0.117408656293409,-0.116242457215294,
-0.102496755730857,-0.095611910182722,-0.0920583897601093,-0.0888709292326105,
-0.074556891706031,-0.0599189423638804,-0.0524290745683954,-0.0472022713413162,
-0.0444388545478162,-0.0293009645371915,-0.0142728755519417,0.),
 .UNSPECIFIED.);
#582=B_SPLINE_CURVE_WITH_KNOTS('',3,(#37019,#37020,#37021,#37022,#37023,
#37024),.UNSPECIFIED.,.F.,.F.,(4,2,4),(0.678296822341137,0.719813557564313,
0.76133029278749),.UNSPECIFIED.);
#583=B_SPLINE_CURVE_WITH_KNOTS('',3,(#37032,#37033,#37034,#37035,#37036,
#37037),.UNSPECIFIED.,.F.,.F.,(4,2,4),(0.678296822341137,0.719813557564313,
0.761330292787489),.UNSPECIFIED.);
#584=B_SPLINE_CURVE_WITH_KNOTS('',3,(#37043,#37044,#37045,#37046,#37047,
#37048),.UNSPECIFIED.,.F.,.F.,(4,2,4),(0.678296822341137,0.719813557564313,
0.76133029278749),.UNSPECIFIED.);
#585=B_SPLINE_CURVE_WITH_KNOTS('',3,(#37054,#37055,#37056,#37057,#37058,
#37059),.UNSPECIFIED.,.F.,.F.,(4,2,4),(0.678296822341137,0.719813557564313,
0.76133029278749),.UNSPECIFIED.);
#586=B_SPLINE_CURVE_WITH_KNOTS('',3,(#37065,#37066,#37067,#37068,#37069,
#37070),.UNSPECIFIED.,.F.,.F.,(4,2,4),(0.678296822341137,0.719813557564313,
0.76133029278749),.UNSPECIFIED.);
#587=B_SPLINE_CURVE_WITH_KNOTS('',3,(#37075,#37076,#37077,#37078,#37079,
#37080),.UNSPECIFIED.,.F.,.F.,(4,2,4),(0.678296822341137,0.719813557564313,
0.76133029278749),.UNSPECIFIED.);
#600=SHAPE_REPRESENTATION_RELATIONSHIP('SRR','None',#37250,#613);
#613=ADVANCED_BREP_SHAPE_REPRESENTATION('',(#639),#37180);
#626=STYLED_ITEM('',(#37380),#639);
#639=MANIFOLD_SOLID_BREP('Body1',#14788);
#688=FACE_BOUND('',#3090,.T.);
#689=FACE_BOUND('',#3095,.T.);
#913=CYLINDRICAL_SURFACE('',#16040,1.215);
#914=CYLINDRICAL_SURFACE('',#16042,1.215);
#915=CYLINDRICAL_SURFACE('',#16043,1.215);
#916=CYLINDRICAL_SURFACE('',#16044,1.215);
#917=CYLINDRICAL_SURFACE('',#16045,1.215);
#918=CYLINDRICAL_SURFACE('',#16046,1.215);
#919=CYLINDRICAL_SURFACE('',#16047,1.215);
#920=CYLINDRICAL_SURFACE('',#16048,1.215);
#921=CYLINDRICAL_SURFACE('',#16049,1.215);
#922=CYLINDRICAL_SURFACE('',#16050,1.215);
#923=CYLINDRICAL_SURFACE('',#16051,1.215);
#924=CYLINDRICAL_SURFACE('',#16052,1.215);
#925=CYLINDRICAL_SURFACE('',#16053,1.215);
#926=CYLINDRICAL_SURFACE('',#16054,1.215);
#927=CYLINDRICAL_SURFACE('',#16055,1.215);
#928=CYLINDRICAL_SURFACE('',#16056,1.215);
#929=CYLINDRICAL_SURFACE('',#16057,1.215);
#930=CYLINDRICAL_SURFACE('',#16058,1.215);
#931=CYLINDRICAL_SURFACE('',#16060,0.95825);
#932=CYLINDRICAL_SURFACE('',#16062,0.95825);
#933=CYLINDRICAL_SURFACE('',#16063,0.95825);
#934=CYLINDRICAL_SURFACE('',#16064,0.95825);
#935=CYLINDRICAL_SURFACE('',#16065,0.95825);
#936=CYLINDRICAL_SURFACE('',#16066,0.95825);
#937=CYLINDRICAL_SURFACE('',#16067,0.95825);
#938=CYLINDRICAL_SURFACE('',#16068,0.95825);
#939=CYLINDRICAL_SURFACE('',#16069,0.95825);
#940=CYLINDRICAL_SURFACE('',#16070,0.95825);
#941=CYLINDRICAL_SURFACE('',#16071,0.95825);
#942=CYLINDRICAL_SURFACE('',#16072,0.95825);
#943=CYLINDRICAL_SURFACE('',#16073,0.95825);
#944=CYLINDRICAL_SURFACE('',#16074,0.95825);
#945=CYLINDRICAL_SURFACE('',#16075,0.95825);
#946=CYLINDRICAL_SURFACE('',#16076,0.95825);
#947=CYLINDRICAL_SURFACE('',#16077,0.95825);
#948=CYLINDRICAL_SURFACE('',#16082,0.95825);
#949=CYLINDRICAL_SURFACE('',#16095,1.215);
#950=CYLINDRICAL_SURFACE('',#16099,2.35);
#1271=CIRCLE('',#16041,1.215);
#1272=CIRCLE('',#16059,1.215);
#1273=CIRCLE('',#16061,0.95825);
#1274=CIRCLE('',#16079,1.215);
#1275=CIRCLE('',#16080,1.215);
#1276=CIRCLE('',#16081,0.95825);
#1277=CIRCLE('',#16084,0.733718498103797);
#1278=CIRCLE('',#16093,1.);
#1279=CIRCLE('',#16096,1.215);
#1280=CIRCLE('',#16098,2.35);
#1281=CIRCLE('',#16100,2.35);
#1282=CIRCLE('',#16101,2.35);
#1366=CONICAL_SURFACE('',#16083,0.375,1.02000541721991);
#1367=CONICAL_SURFACE('',#16094,1.125,0.785398163397448);
#2155=FACE_OUTER_BOUND('',#3043,.T.);
#2156=FACE_OUTER_BOUND('',#3044,.T.);
#2157=FACE_OUTER_BOUND('',#3045,.T.);
#2158=FACE_OUTER_BOUND('',#3046,.T.);
#2159=FACE_OUTER_BOUND('',#3047,.T.);
#2160=FACE_OUTER_BOUND('',#3048,.T.);
#2161=FACE_OUTER_BOUND('',#3049,.T.);
#2162=FACE_OUTER_BOUND('',#3050,.T.);
#2163=FACE_OUTER_BOUND('',#3051,.T.);
#2164=FACE_OUTER_BOUND('',#3052,.T.);
#2165=FACE_OUTER_BOUND('',#3053,.T.);
#2166=FACE_OUTER_BOUND('',#3054,.T.);
#2167=FACE_OUTER_BOUND('',#3055,.T.);
#2168=FACE_OUTER_BOUND('',#3056,.T.);
#2169=FACE_OUTER_BOUND('',#3057,.T.);
#2170=FACE_OUTER_BOUND('',#3058,.T.);
#2171=FACE_OUTER_BOUND('',#3059,.T.);
#2172=FACE_OUTER_BOUND('',#3060,.T.);
#2173=FACE_OUTER_BOUND('',#3061,.T.);
#2174=FACE_OUTER_BOUND('',#3062,.T.);
#2175=FACE_OUTER_BOUND('',#3063,.T.);
#2176=FACE_OUTER_BOUND('',#3064,.T.);
#2177=FACE_OUTER_BOUND('',#3065,.T.);
#2178=FACE_OUTER_BOUND('',#3066,.T.);
#2179=FACE_OUTER_BOUND('',#3067,.T.);
#2180=FACE_OUTER_BOUND('',#3068,.T.);
#2181=FACE_OUTER_BOUND('',#3069,.T.);
#2182=FACE_OUTER_BOUND('',#3070,.T.);
#2183=FACE_OUTER_BOUND('',#3071,.T.);
#2184=FACE_OUTER_BOUND('',#3072,.T.);
#2185=FACE_OUTER_BOUND('',#3073,.T.);
#2186=FACE_OUTER_BOUND('',#3074,.T.);
#2187=FACE_OUTER_BOUND('',#3075,.T.);
#2188=FACE_OUTER_BOUND('',#3076,.T.);
#2189=FACE_OUTER_BOUND('',#3077,.T.);
#2190=FACE_OUTER_BOUND('',#3078,.T.);
#2191=FACE_OUTER_BOUND('',#3079,.T.);
#2192=FACE_OUTER_BOUND('',#3080,.T.);
#2193=FACE_OUTER_BOUND('',#3081,.T.);
#2194=FACE_OUTER_BOUND('',#3082,.T.);
#2195=FACE_OUTER_BOUND('',#3083,.T.);
#2196=FACE_OUTER_BOUND('',#3084,.T.);
#2197=FACE_OUTER_BOUND('',#3085,.T.);
#2198=FACE_OUTER_BOUND('',#3086,.T.);
#2199=FACE_OUTER_BOUND('',#3087,.T.);
#2200=FACE_OUTER_BOUND('',#3088,.T.);
#2201=FACE_OUTER_BOUND('',#3089,.T.);
#2202=FACE_OUTER_BOUND('',#3091,.T.);
#2203=FACE_OUTER_BOUND('',#3092,.T.);
#2204=FACE_OUTER_BOUND('',#3093,.T.);
#2205=FACE_OUTER_BOUND('',#3094,.T.);
#2206=FACE_OUTER_BOUND('',#3096,.T.);
#2207=FACE_OUTER_BOUND('',#3097,.T.);
#3043=EDGE_LOOP('',(#13167,#13168,#13169,#13170));
#3044=EDGE_LOOP('',(#13171,#13172,#13173,#13174));
#3045=EDGE_LOOP('',(#13175,#13176,#13177,#13178));
#3046=EDGE_LOOP('',(#13179,#13180,#13181,#13182));
#3047=EDGE_LOOP('',(#13183,#13184,#13185,#13186));
#3048=EDGE_LOOP('',(#13187,#13188,#13189,#13190));
#3049=EDGE_LOOP('',(#13191,#13192,#13193,#13194));
#3050=EDGE_LOOP('',(#13195,#13196,#13197,#13198));
#3051=EDGE_LOOP('',(#13199,#13200,#13201,#13202));
#3052=EDGE_LOOP('',(#13203,#13204,#13205,#13206));
#3053=EDGE_LOOP('',(#13207,#13208,#13209,#13210));
#3054=EDGE_LOOP('',(#13211,#13212,#13213,#13214));
#3055=EDGE_LOOP('',(#13215,#13216,#13217,#13218));
#3056=EDGE_LOOP('',(#13219,#13220,#13221,#13222));
#3057=EDGE_LOOP('',(#13223,#13224,#13225,#13226));
#3058=EDGE_LOOP('',(#13227,#13228,#13229,#13230));
#3059=EDGE_LOOP('',(#13231,#13232,#13233,#13234));
#3060=EDGE_LOOP('',(#13235,#13236,#13237,#13238,#13239));
#3061=EDGE_LOOP('',(#13240,#13241,#13242,#13243));
#3062=EDGE_LOOP('',(#13244,#13245,#13246,#13247));
#3063=EDGE_LOOP('',(#13248,#13249,#13250,#13251));
#3064=EDGE_LOOP('',(#13252,#13253,#13254,#13255));
#3065=EDGE_LOOP('',(#13256,#13257,#13258,#13259));
#3066=EDGE_LOOP('',(#13260,#13261,#13262,#13263));
#3067=EDGE_LOOP('',(#13264,#13265,#13266,#13267));
#3068=EDGE_LOOP('',(#13268,#13269,#13270,#13271));
#3069=EDGE_LOOP('',(#13272,#13273,#13274,#13275));
#3070=EDGE_LOOP('',(#13276,#13277,#13278,#13279));
#3071=EDGE_LOOP('',(#13280,#13281,#13282,#13283));
#3072=EDGE_LOOP('',(#13284,#13285,#13286,#13287));
#3073=EDGE_LOOP('',(#13288,#13289,#13290,#13291));
#3074=EDGE_LOOP('',(#13292,#13293,#13294,#13295));
#3075=EDGE_LOOP('',(#13296,#13297,#13298,#13299));
#3076=EDGE_LOOP('',(#13300,#13301,#13302,#13303));
#3077=EDGE_LOOP('',(#13304,#13305,#13306,#13307));
#3078=EDGE_LOOP('',(#13308,#13309,#13310,#13311,#13312,#13313,#13314,#13315,
#13316,#13317,#13318,#13319,#13320,#13321,#13322,#13323,#13324,#13325,#13326,
#13327,#13328,#13329,#13330,#13331,#13332,#13333,#13334,#13335,#13336,#13337,
#13338,#13339,#13340,#13341,#13342,#13343,#13344,#13345,#13346));
#3079=EDGE_LOOP('',(#13347,#13348,#13349,#13350,#13351));
#3080=EDGE_LOOP('',(#13352,#13353,#13354,#13355));
#3081=EDGE_LOOP('',(#13356,#13357,#13358,#13359,#13360,#13361,#13362,#13363,
#13364,#13365,#13366,#13367,#13368,#13369,#13370,#13371,#13372,#13373,#13374,
#13375,#13376,#13377,#13378,#13379,#13380,#13381,#13382,#13383,#13384,#13385,
#13386,#13387,#13388,#13389,#13390,#13391,#13392,#13393));
#3082=EDGE_LOOP('',(#13394,#13395,#13396));
#3083=EDGE_LOOP('',(#13397,#13398,#13399,#13400));
#3084=EDGE_LOOP('',(#13401,#13402,#13403,#13404));
#3085=EDGE_LOOP('',(#13405,#13406,#13407,#13408));
#3086=EDGE_LOOP('',(#13409,#13410,#13411,#13412));
#3087=EDGE_LOOP('',(#13413,#13414,#13415,#13416));
#3088=EDGE_LOOP('',(#13417,#13418,#13419,#13420));
#3089=EDGE_LOOP('',(#13421,#13422,#13423,#13424,#13425,#13426));
#3090=EDGE_LOOP('',(#13427));
#3091=EDGE_LOOP('',(#13428));
#3092=EDGE_LOOP('',(#13429,#13430,#13431,#13432,#13433,#13434));
#3093=EDGE_LOOP('',(#13435,#13436,#13437));
#3094=EDGE_LOOP('',(#13438));
#3095=EDGE_LOOP('',(#13439,#13440,#13441,#13442,#13443));
#3096=EDGE_LOOP('',(#13444,#13445,#13446,#13447,#13448));
#3097=EDGE_LOOP('',(#13449,#13450,#13451,#13452,#13453,#13454,#13455,#13456,
#13457,#13458));
#3202=(
BOUNDED_CURVE()
B_SPLINE_CURVE(2,(#37126,#37127,#37128),.UNSPECIFIED.,.F.,.F.)
B_SPLINE_CURVE_WITH_KNOTS((3,3),(-1.33896509897879,-0.513408172091738),
 .UNSPECIFIED.)
CURVE()
GEOMETRIC_REPRESENTATION_ITEM()
RATIONAL_B_SPLINE_CURVE((0.98929230069637,0.910813429578529,1.))
REPRESENTATION_ITEM('')
);
#4392=LINE('',#34461,#5631);
#4393=LINE('',#34485,#5632);
#4394=LINE('',#34533,#5633);
#4395=LINE('',#34581,#5634);
#4396=LINE('',#34632,#5635);
#4397=LINE('',#34683,#5636);
#4398=LINE('',#34731,#5637);
#4399=LINE('',#34779,#5638);
#4400=LINE('',#34833,#5639);
#4401=LINE('',#34881,#5640);
#4402=LINE('',#34929,#5641);
#4403=LINE('',#34983,#5642);
#4404=LINE('',#35031,#5643);
#4405=LINE('',#35079,#5644);
#4406=LINE('',#35127,#5645);
#4407=LINE('',#35181,#5646);
#4408=LINE('',#35229,#5647);
#4409=LINE('',#35277,#5648);
#4410=LINE('',#35330,#5649);
#4411=LINE('',#35351,#5650);
#4412=LINE('',#35376,#5651);
#4413=LINE('',#35400,#5652);
#4414=LINE('',#35425,#5653);
#4415=LINE('',#35450,#5654);
#4416=LINE('',#35474,#5655);
#4417=LINE('',#35498,#5656);
#4418=LINE('',#35523,#5657);
#4419=LINE('',#35548,#5658);
#4420=LINE('',#35572,#5659);
#4421=LINE('',#35597,#5660);
#4422=LINE('',#35622,#5661);
#4423=LINE('',#35646,#5662);
#4424=LINE('',#35671,#5663);
#4425=LINE('',#35695,#5664);
#4426=LINE('',#35720,#5665);
#4427=LINE('',#37014,#5666);
#4428=LINE('',#37026,#5667);
#4429=LINE('',#37028,#5668);
#4430=LINE('',#37029,#5669);
#4431=LINE('',#37039,#5670);
#4432=LINE('',#37040,#5671);
#4433=LINE('',#37050,#5672);
#4434=LINE('',#37051,#5673);
#4435=LINE('',#37061,#5674);
#4436=LINE('',#37062,#5675);
#4437=LINE('',#37072,#5676);
#4438=LINE('',#37073,#5677);
#4439=LINE('',#37081,#5678);
#4440=LINE('',#37087,#5679);
#4441=LINE('',#37097,#5680);
#5631=VECTOR('',#19530,1.25);
#5632=VECTOR('',#19535,1.25);
#5633=VECTOR('',#19538,1.25);
#5634=VECTOR('',#19541,1.25);
#5635=VECTOR('',#19544,1.25);
#5636=VECTOR('',#19547,1.25);
#5637=VECTOR('',#19550,1.25);
#5638=VECTOR('',#19553,1.25);
#5639=VECTOR('',#19556,1.25);
#5640=VECTOR('',#19559,1.25);
#5641=VECTOR('',#19562,1.25);
#5642=VECTOR('',#19565,1.25);
#5643=VECTOR('',#19568,1.25);
#5644=VECTOR('',#19571,1.25);
#5645=VECTOR('',#19574,1.25);
#5646=VECTOR('',#19577,1.25);
#5647=VECTOR('',#19580,1.25);
#5648=VECTOR('',#19583,1.25);
#5649=VECTOR('',#19588,0.95825);
#5650=VECTOR('',#19593,0.95825);
#5651=VECTOR('',#19596,0.95825);
#5652=VECTOR('',#19599,0.95825);
#5653=VECTOR('',#19602,0.95825);
#5654=VECTOR('',#19605,0.95825);
#5655=VECTOR('',#19608,0.95825);
#5656=VECTOR('',#19611,0.95825);
#5657=VECTOR('',#19614,0.95825);
#5658=VECTOR('',#19617,0.95825);
#5659=VECTOR('',#19620,0.95825);
#5660=VECTOR('',#19623,0.95825);
#5661=VECTOR('',#19626,0.95825);
#5662=VECTOR('',#19629,0.95825);
#5663=VECTOR('',#19632,0.95825);
#5664=VECTOR('',#19635,0.95825);
#5665=VECTOR('',#19638,0.95825);
#5666=VECTOR('',#19651,0.375);
#5667=VECTOR('',#19656,10.);
#5668=VECTOR('',#19657,10.);
#5669=VECTOR('',#19658,10.);
#5670=VECTOR('',#19661,10.);
#5671=VECTOR('',#19662,10.);
#5672=VECTOR('',#19665,10.);
#5673=VECTOR('',#19666,10.);
#5674=VECTOR('',#19669,10.);
#5675=VECTOR('',#19670,10.);
#5676=VECTOR('',#19673,10.);
#5677=VECTOR('',#19674,10.);
#5678=VECTOR('',#19677,10.);
#5679=VECTOR('',#19686,1.125);
#5680=VECTOR('',#19699,2.35);
#6930=VERTEX_POINT('',#34459);
#6931=VERTEX_POINT('',#34460);
#6932=VERTEX_POINT('',#34462);
#6933=VERTEX_POINT('',#34473);
#6934=VERTEX_POINT('',#34483);
#6935=VERTEX_POINT('',#34484);
#6936=VERTEX_POINT('',#34531);
#6937=VERTEX_POINT('',#34532);
#6938=VERTEX_POINT('',#34579);
#6939=VERTEX_POINT('',#34580);
#6940=VERTEX_POINT('',#34630);
#6941=VERTEX_POINT('',#34631);
#6942=VERTEX_POINT('',#34681);
#6943=VERTEX_POINT('',#34682);
#6944=VERTEX_POINT('',#34729);
#6945=VERTEX_POINT('',#34730);
#6946=VERTEX_POINT('',#34777);
#6947=VERTEX_POINT('',#34778);
#6948=VERTEX_POINT('',#34831);
#6949=VERTEX_POINT('',#34832);
#6950=VERTEX_POINT('',#34879);
#6951=VERTEX_POINT('',#34880);
#6952=VERTEX_POINT('',#34927);
#6953=VERTEX_POINT('',#34928);
#6954=VERTEX_POINT('',#34981);
#6955=VERTEX_POINT('',#34982);
#6956=VERTEX_POINT('',#35029);
#6957=VERTEX_POINT('',#35030);
#6958=VERTEX_POINT('',#35077);
#6959=VERTEX_POINT('',#35078);
#6960=VERTEX_POINT('',#35125);
#6961=VERTEX_POINT('',#35126);
#6962=VERTEX_POINT('',#35179);
#6963=VERTEX_POINT('',#35180);
#6964=VERTEX_POINT('',#35227);
#6965=VERTEX_POINT('',#35228);
#6966=VERTEX_POINT('',#35275);
#6967=VERTEX_POINT('',#35276);
#6968=VERTEX_POINT('',#35278);
#6969=VERTEX_POINT('',#35328);
#6970=VERTEX_POINT('',#35329);
#6971=VERTEX_POINT('',#35331);
#6972=VERTEX_POINT('',#35340);
#6973=VERTEX_POINT('',#35349);
#6974=VERTEX_POINT('',#35350);
#6975=VERTEX_POINT('',#35374);
#6976=VERTEX_POINT('',#35375);
#6977=VERTEX_POINT('',#35398);
#6978=VERTEX_POINT('',#35399);
#6979=VERTEX_POINT('',#35423);
#6980=VERTEX_POINT('',#35424);
#6981=VERTEX_POINT('',#35448);
#6982=VERTEX_POINT('',#35449);
#6983=VERTEX_POINT('',#35472);
#6984=VERTEX_POINT('',#35473);
#6985=VERTEX_POINT('',#35496);
#6986=VERTEX_POINT('',#35497);
#6987=VERTEX_POINT('',#35521);
#6988=VERTEX_POINT('',#35522);
#6989=VERTEX_POINT('',#35546);
#6990=VERTEX_POINT('',#35547);
#6991=VERTEX_POINT('',#35570);
#6992=VERTEX_POINT('',#35571);
#6993=VERTEX_POINT('',#35595);
#6994=VERTEX_POINT('',#35596);
#6995=VERTEX_POINT('',#35620);
#6996=VERTEX_POINT('',#35621);
#6997=VERTEX_POINT('',#35644);
#6998=VERTEX_POINT('',#35645);
#6999=VERTEX_POINT('',#35669);
#7000=VERTEX_POINT('',#35670);
#7001=VERTEX_POINT('',#35693);
#7002=VERTEX_POINT('',#35694);
#7003=VERTEX_POINT('',#35718);
#7004=VERTEX_POINT('',#35719);
#7005=VERTEX_POINT('',#36197);
#7006=VERTEX_POINT('',#36284);
#7007=VERTEX_POINT('',#36377);
#7008=VERTEX_POINT('',#36380);
#7009=VERTEX_POINT('',#37012);
#7010=VERTEX_POINT('',#37013);
#7011=VERTEX_POINT('',#37017);
#7012=VERTEX_POINT('',#37018);
#7013=VERTEX_POINT('',#37025);
#7014=VERTEX_POINT('',#37027);
#7015=VERTEX_POINT('',#37031);
#7016=VERTEX_POINT('',#37038);
#7017=VERTEX_POINT('',#37042);
#7018=VERTEX_POINT('',#37049);
#7019=VERTEX_POINT('',#37053);
#7020=VERTEX_POINT('',#37060);
#7021=VERTEX_POINT('',#37064);
#7022=VERTEX_POINT('',#37071);
#7023=VERTEX_POINT('',#37084);
#7024=VERTEX_POINT('',#37091);
#7025=VERTEX_POINT('',#37094);
#7026=VERTEX_POINT('',#37095);
#9025=EDGE_CURVE('',#6930,#6931,#4392,.T.);
#9026=EDGE_CURVE('',#6930,#6932,#505,.T.);
#9027=EDGE_CURVE('',#6932,#6933,#1271,.T.);
#9028=EDGE_CURVE('',#6933,#6931,#506,.T.);
#9029=EDGE_CURVE('',#6934,#6935,#4393,.T.);
#9030=EDGE_CURVE('',#6934,#6930,#507,.T.);
#9031=EDGE_CURVE('',#6931,#6935,#508,.T.);
#9032=EDGE_CURVE('',#6936,#6937,#4394,.T.);
#9033=EDGE_CURVE('',#6936,#6934,#509,.T.);
#9034=EDGE_CURVE('',#6935,#6937,#510,.T.);
#9035=EDGE_CURVE('',#6938,#6939,#4395,.T.);
#9036=EDGE_CURVE('',#6938,#6936,#511,.T.);
#9037=EDGE_CURVE('',#6937,#6939,#512,.T.);
#9038=EDGE_CURVE('',#6940,#6941,#4396,.T.);
#9039=EDGE_CURVE('',#6940,#6938,#513,.T.);
#9040=EDGE_CURVE('',#6939,#6941,#514,.T.);
#9041=EDGE_CURVE('',#6942,#6943,#4397,.T.);
#9042=EDGE_CURVE('',#6942,#6940,#515,.T.);
#9043=EDGE_CURVE('',#6941,#6943,#516,.T.);
#9044=EDGE_CURVE('',#6944,#6945,#4398,.T.);
#9045=EDGE_CURVE('',#6944,#6942,#517,.T.);
#9046=EDGE_CURVE('',#6943,#6945,#518,.T.);
#9047=EDGE_CURVE('',#6946,#6947,#4399,.T.);
#9048=EDGE_CURVE('',#6946,#6944,#519,.T.);
#9049=EDGE_CURVE('',#6945,#6947,#520,.T.);
#9050=EDGE_CURVE('',#6948,#6949,#4400,.T.);
#9051=EDGE_CURVE('',#6948,#6946,#521,.T.);
#9052=EDGE_CURVE('',#6947,#6949,#522,.T.);
#9053=EDGE_CURVE('',#6950,#6951,#4401,.T.);
#9054=EDGE_CURVE('',#6950,#6948,#523,.T.);
#9055=EDGE_CURVE('',#6949,#6951,#524,.T.);
#9056=EDGE_CURVE('',#6952,#6953,#4402,.T.);
#9057=EDGE_CURVE('',#6952,#6950,#525,.T.);
#9058=EDGE_CURVE('',#6951,#6953,#526,.T.);
#9059=EDGE_CURVE('',#6954,#6955,#4403,.T.);
#9060=EDGE_CURVE('',#6954,#6952,#527,.T.);
#9061=EDGE_CURVE('',#6953,#6955,#528,.T.);
#9062=EDGE_CURVE('',#6956,#6957,#4404,.T.);
#9063=EDGE_CURVE('',#6956,#6954,#529,.T.);
#9064=EDGE_CURVE('',#6955,#6957,#530,.T.);
#9065=EDGE_CURVE('',#6958,#6959,#4405,.T.);
#9066=EDGE_CURVE('',#6958,#6956,#531,.T.);
#9067=EDGE_CURVE('',#6957,#6959,#532,.T.);
#9068=EDGE_CURVE('',#6960,#6961,#4406,.T.);
#9069=EDGE_CURVE('',#6960,#6958,#533,.T.);
#9070=EDGE_CURVE('',#6959,#6961,#534,.T.);
#9071=EDGE_CURVE('',#6962,#6963,#4407,.T.);
#9072=EDGE_CURVE('',#6962,#6960,#535,.T.);
#9073=EDGE_CURVE('',#6961,#6963,#536,.T.);
#9074=EDGE_CURVE('',#6964,#6965,#4408,.T.);
#9075=EDGE_CURVE('',#6964,#6962,#537,.T.);
#9076=EDGE_CURVE('',#6963,#6965,#538,.T.);
#9077=EDGE_CURVE('',#6966,#6967,#4409,.T.);
#9078=EDGE_CURVE('',#6968,#6966,#1272,.T.);
#9079=EDGE_CURVE('',#6968,#6964,#539,.T.);
#9080=EDGE_CURVE('',#6965,#6967,#540,.T.);
#9081=EDGE_CURVE('',#6969,#6970,#4410,.T.);
#9082=EDGE_CURVE('',#6969,#6971,#541,.T.);
#9083=EDGE_CURVE('',#6972,#6971,#1273,.T.);
#9084=EDGE_CURVE('',#6970,#6972,#542,.T.);
#9085=EDGE_CURVE('',#6973,#6974,#4411,.T.);
#9086=EDGE_CURVE('',#6973,#6969,#543,.T.);
#9087=EDGE_CURVE('',#6974,#6970,#544,.T.);
#9088=EDGE_CURVE('',#6975,#6976,#4412,.T.);
#9089=EDGE_CURVE('',#6975,#6973,#545,.T.);
#9090=EDGE_CURVE('',#6976,#6974,#546,.T.);
#9091=EDGE_CURVE('',#6977,#6978,#4413,.T.);
#9092=EDGE_CURVE('',#6977,#6975,#547,.T.);
#9093=EDGE_CURVE('',#6978,#6976,#548,.T.);
#9094=EDGE_CURVE('',#6979,#6980,#4414,.T.);
#9095=EDGE_CURVE('',#6979,#6977,#549,.T.);
#9096=EDGE_CURVE('',#6980,#6978,#550,.T.);
#9097=EDGE_CURVE('',#6981,#6982,#4415,.T.);
#9098=EDGE_CURVE('',#6981,#6979,#551,.T.);
#9099=EDGE_CURVE('',#6982,#6980,#552,.T.);
#9100=EDGE_CURVE('',#6983,#6984,#4416,.T.);
#9101=EDGE_CURVE('',#6983,#6981,#553,.T.);
#9102=EDGE_CURVE('',#6984,#6982,#554,.T.);
#9103=EDGE_CURVE('',#6985,#6986,#4417,.T.);
#9104=EDGE_CURVE('',#6985,#6983,#555,.T.);
#9105=EDGE_CURVE('',#6986,#6984,#556,.T.);
#9106=EDGE_CURVE('',#6987,#6988,#4418,.T.);
#9107=EDGE_CURVE('',#6987,#6985,#557,.T.);
#9108=EDGE_CURVE('',#6988,#6986,#558,.T.);
#9109=EDGE_CURVE('',#6989,#6990,#4419,.T.);
#9110=EDGE_CURVE('',#6989,#6987,#559,.T.);
#9111=EDGE_CURVE('',#6990,#6988,#560,.T.);
#9112=EDGE_CURVE('',#6991,#6992,#4420,.T.);
#9113=EDGE_CURVE('',#6991,#6989,#561,.T.);
#9114=EDGE_CURVE('',#6992,#6990,#562,.T.);
#9115=EDGE_CURVE('',#6993,#6994,#4421,.T.);
#9116=EDGE_CURVE('',#6993,#6991,#563,.T.);
#9117=EDGE_CURVE('',#6994,#6992,#564,.T.);
#9118=EDGE_CURVE('',#6995,#6996,#4422,.T.);
#9119=EDGE_CURVE('',#6995,#6993,#565,.T.);
#9120=EDGE_CURVE('',#6996,#6994,#566,.T.);
#9121=EDGE_CURVE('',#6997,#6998,#4423,.T.);
#9122=EDGE_CURVE('',#6997,#6995,#567,.T.);
#9123=EDGE_CURVE('',#6998,#6996,#568,.T.);
#9124=EDGE_CURVE('',#6999,#7000,#4424,.T.);
#9125=EDGE_CURVE('',#6999,#6997,#569,.T.);
#9126=EDGE_CURVE('',#7000,#6998,#570,.T.);
#9127=EDGE_CURVE('',#7001,#7002,#4425,.T.);
#9128=EDGE_CURVE('',#7001,#6999,#571,.T.);
#9129=EDGE_CURVE('',#7002,#7000,#572,.T.);
#9130=EDGE_CURVE('',#7003,#7004,#4426,.T.);
#9131=EDGE_CURVE('',#7003,#7001,#573,.T.);
#9132=EDGE_CURVE('',#7004,#7002,#574,.T.);
#9133=EDGE_CURVE('',#7005,#6972,#575,.T.);
#9134=EDGE_CURVE('',#6967,#7005,#576,.T.);
#9135=EDGE_CURVE('',#7006,#6933,#577,.T.);
#9136=EDGE_CURVE('',#7006,#7004,#578,.T.);
#9137=EDGE_CURVE('',#6933,#7007,#1274,.T.);
#9138=EDGE_CURVE('',#7007,#6932,#1275,.T.);
#9139=EDGE_CURVE('',#6932,#7008,#579,.T.);
#9140=EDGE_CURVE('',#7008,#7006,#1276,.T.);
#9141=EDGE_CURVE('',#7008,#7003,#580,.T.);
#9142=EDGE_CURVE('',#6971,#6968,#581,.T.);
#9143=EDGE_CURVE('',#7009,#7010,#4427,.T.);
#9144=EDGE_CURVE('',#7010,#7010,#1277,.T.);
#9145=EDGE_CURVE('',#7011,#7012,#582,.T.);
#9146=EDGE_CURVE('',#7011,#7013,#4428,.T.);
#9147=EDGE_CURVE('',#7013,#7014,#4429,.T.);
#9148=EDGE_CURVE('',#7012,#7014,#4430,.T.);
#9149=EDGE_CURVE('',#7012,#7015,#583,.T.);
#9150=EDGE_CURVE('',#7014,#7016,#4431,.T.);
#9151=EDGE_CURVE('',#7015,#7016,#4432,.T.);
#9152=EDGE_CURVE('',#7015,#7017,#584,.T.);
#9153=EDGE_CURVE('',#7016,#7018,#4433,.T.);
#9154=EDGE_CURVE('',#7017,#7018,#4434,.T.);
#9155=EDGE_CURVE('',#7017,#7019,#585,.T.);
#9156=EDGE_CURVE('',#7018,#7020,#4435,.T.);
#9157=EDGE_CURVE('',#7019,#7020,#4436,.T.);
#9158=EDGE_CURVE('',#7021,#7011,#586,.T.);
#9159=EDGE_CURVE('',#7021,#7022,#4437,.T.);
#9160=EDGE_CURVE('',#7022,#7013,#4438,.T.);
#9161=EDGE_CURVE('',#7019,#7021,#587,.T.);
#9162=EDGE_CURVE('',#7020,#7022,#4439,.T.);
#9163=EDGE_CURVE('',#7023,#7023,#1278,.T.);
#9164=EDGE_CURVE('',#7007,#7023,#4440,.T.);
#9165=EDGE_CURVE('',#6966,#7005,#1279,.T.);
#9166=EDGE_CURVE('',#7024,#7024,#1280,.T.);
#9167=EDGE_CURVE('',#7025,#7026,#1281,.T.);
#9168=EDGE_CURVE('',#7025,#7024,#4441,.T.);
#9169=EDGE_CURVE('',#7026,#7025,#1282,.T.);
#9170=EDGE_CURVE('',#7017,#7026,#3202,.T.);
#13167=ORIENTED_EDGE('',*,*,#9025,.F.);
#13168=ORIENTED_EDGE('',*,*,#9026,.T.);
#13169=ORIENTED_EDGE('',*,*,#9027,.T.);
#13170=ORIENTED_EDGE('',*,*,#9028,.T.);
#13171=ORIENTED_EDGE('',*,*,#9029,.F.);
#13172=ORIENTED_EDGE('',*,*,#9030,.T.);
#13173=ORIENTED_EDGE('',*,*,#9025,.T.);
#13174=ORIENTED_EDGE('',*,*,#9031,.T.);
#13175=ORIENTED_EDGE('',*,*,#9032,.F.);
#13176=ORIENTED_EDGE('',*,*,#9033,.T.);
#13177=ORIENTED_EDGE('',*,*,#9029,.T.);
#13178=ORIENTED_EDGE('',*,*,#9034,.T.);
#13179=ORIENTED_EDGE('',*,*,#9035,.F.);
#13180=ORIENTED_EDGE('',*,*,#9036,.T.);
#13181=ORIENTED_EDGE('',*,*,#9032,.T.);
#13182=ORIENTED_EDGE('',*,*,#9037,.T.);
#13183=ORIENTED_EDGE('',*,*,#9038,.F.);
#13184=ORIENTED_EDGE('',*,*,#9039,.T.);
#13185=ORIENTED_EDGE('',*,*,#9035,.T.);
#13186=ORIENTED_EDGE('',*,*,#9040,.T.);
#13187=ORIENTED_EDGE('',*,*,#9041,.F.);
#13188=ORIENTED_EDGE('',*,*,#9042,.T.);
#13189=ORIENTED_EDGE('',*,*,#9038,.T.);
#13190=ORIENTED_EDGE('',*,*,#9043,.T.);
#13191=ORIENTED_EDGE('',*,*,#9044,.F.);
#13192=ORIENTED_EDGE('',*,*,#9045,.T.);
#13193=ORIENTED_EDGE('',*,*,#9041,.T.);
#13194=ORIENTED_EDGE('',*,*,#9046,.T.);
#13195=ORIENTED_EDGE('',*,*,#9047,.F.);
#13196=ORIENTED_EDGE('',*,*,#9048,.T.);
#13197=ORIENTED_EDGE('',*,*,#9044,.T.);
#13198=ORIENTED_EDGE('',*,*,#9049,.T.);
#13199=ORIENTED_EDGE('',*,*,#9050,.F.);
#13200=ORIENTED_EDGE('',*,*,#9051,.T.);
#13201=ORIENTED_EDGE('',*,*,#9047,.T.);
#13202=ORIENTED_EDGE('',*,*,#9052,.T.);
#13203=ORIENTED_EDGE('',*,*,#9053,.F.);
#13204=ORIENTED_EDGE('',*,*,#9054,.T.);
#13205=ORIENTED_EDGE('',*,*,#9050,.T.);
#13206=ORIENTED_EDGE('',*,*,#9055,.T.);
#13207=ORIENTED_EDGE('',*,*,#9056,.F.);
#13208=ORIENTED_EDGE('',*,*,#9057,.T.);
#13209=ORIENTED_EDGE('',*,*,#9053,.T.);
#13210=ORIENTED_EDGE('',*,*,#9058,.T.);
#13211=ORIENTED_EDGE('',*,*,#9059,.F.);
#13212=ORIENTED_EDGE('',*,*,#9060,.T.);
#13213=ORIENTED_EDGE('',*,*,#9056,.T.);
#13214=ORIENTED_EDGE('',*,*,#9061,.T.);
#13215=ORIENTED_EDGE('',*,*,#9062,.F.);
#13216=ORIENTED_EDGE('',*,*,#9063,.T.);
#13217=ORIENTED_EDGE('',*,*,#9059,.T.);
#13218=ORIENTED_EDGE('',*,*,#9064,.T.);
#13219=ORIENTED_EDGE('',*,*,#9065,.F.);
#13220=ORIENTED_EDGE('',*,*,#9066,.T.);
#13221=ORIENTED_EDGE('',*,*,#9062,.T.);
#13222=ORIENTED_EDGE('',*,*,#9067,.T.);
#13223=ORIENTED_EDGE('',*,*,#9068,.F.);
#13224=ORIENTED_EDGE('',*,*,#9069,.T.);
#13225=ORIENTED_EDGE('',*,*,#9065,.T.);
#13226=ORIENTED_EDGE('',*,*,#9070,.T.);
#13227=ORIENTED_EDGE('',*,*,#9071,.F.);
#13228=ORIENTED_EDGE('',*,*,#9072,.T.);
#13229=ORIENTED_EDGE('',*,*,#9068,.T.);
#13230=ORIENTED_EDGE('',*,*,#9073,.T.);
#13231=ORIENTED_EDGE('',*,*,#9074,.F.);
#13232=ORIENTED_EDGE('',*,*,#9075,.T.);
#13233=ORIENTED_EDGE('',*,*,#9071,.T.);
#13234=ORIENTED_EDGE('',*,*,#9076,.T.);
#13235=ORIENTED_EDGE('',*,*,#9077,.F.);
#13236=ORIENTED_EDGE('',*,*,#9078,.F.);
#13237=ORIENTED_EDGE('',*,*,#9079,.T.);
#13238=ORIENTED_EDGE('',*,*,#9074,.T.);
#13239=ORIENTED_EDGE('',*,*,#9080,.T.);
#13240=ORIENTED_EDGE('',*,*,#9081,.F.);
#13241=ORIENTED_EDGE('',*,*,#9082,.T.);
#13242=ORIENTED_EDGE('',*,*,#9083,.F.);
#13243=ORIENTED_EDGE('',*,*,#9084,.F.);
#13244=ORIENTED_EDGE('',*,*,#9085,.F.);
#13245=ORIENTED_EDGE('',*,*,#9086,.T.);
#13246=ORIENTED_EDGE('',*,*,#9081,.T.);
#13247=ORIENTED_EDGE('',*,*,#9087,.F.);
#13248=ORIENTED_EDGE('',*,*,#9088,.F.);
#13249=ORIENTED_EDGE('',*,*,#9089,.T.);
#13250=ORIENTED_EDGE('',*,*,#9085,.T.);
#13251=ORIENTED_EDGE('',*,*,#9090,.F.);
#13252=ORIENTED_EDGE('',*,*,#9091,.F.);
#13253=ORIENTED_EDGE('',*,*,#9092,.T.);
#13254=ORIENTED_EDGE('',*,*,#9088,.T.);
#13255=ORIENTED_EDGE('',*,*,#9093,.F.);
#13256=ORIENTED_EDGE('',*,*,#9094,.F.);
#13257=ORIENTED_EDGE('',*,*,#9095,.T.);
#13258=ORIENTED_EDGE('',*,*,#9091,.T.);
#13259=ORIENTED_EDGE('',*,*,#9096,.F.);
#13260=ORIENTED_EDGE('',*,*,#9097,.F.);
#13261=ORIENTED_EDGE('',*,*,#9098,.T.);
#13262=ORIENTED_EDGE('',*,*,#9094,.T.);
#13263=ORIENTED_EDGE('',*,*,#9099,.F.);
#13264=ORIENTED_EDGE('',*,*,#9100,.F.);
#13265=ORIENTED_EDGE('',*,*,#9101,.T.);
#13266=ORIENTED_EDGE('',*,*,#9097,.T.);
#13267=ORIENTED_EDGE('',*,*,#9102,.F.);
#13268=ORIENTED_EDGE('',*,*,#9103,.F.);
#13269=ORIENTED_EDGE('',*,*,#9104,.T.);
#13270=ORIENTED_EDGE('',*,*,#9100,.T.);
#13271=ORIENTED_EDGE('',*,*,#9105,.F.);
#13272=ORIENTED_EDGE('',*,*,#9106,.F.);
#13273=ORIENTED_EDGE('',*,*,#9107,.T.);
#13274=ORIENTED_EDGE('',*,*,#9103,.T.);
#13275=ORIENTED_EDGE('',*,*,#9108,.F.);
#13276=ORIENTED_EDGE('',*,*,#9109,.F.);
#13277=ORIENTED_EDGE('',*,*,#9110,.T.);
#13278=ORIENTED_EDGE('',*,*,#9106,.T.);
#13279=ORIENTED_EDGE('',*,*,#9111,.F.);
#13280=ORIENTED_EDGE('',*,*,#9112,.F.);
#13281=ORIENTED_EDGE('',*,*,#9113,.T.);
#13282=ORIENTED_EDGE('',*,*,#9109,.T.);
#13283=ORIENTED_EDGE('',*,*,#9114,.F.);
#13284=ORIENTED_EDGE('',*,*,#9115,.F.);
#13285=ORIENTED_EDGE('',*,*,#9116,.T.);
#13286=ORIENTED_EDGE('',*,*,#9112,.T.);
#13287=ORIENTED_EDGE('',*,*,#9117,.F.);
#13288=ORIENTED_EDGE('',*,*,#9118,.F.);
#13289=ORIENTED_EDGE('',*,*,#9119,.T.);
#13290=ORIENTED_EDGE('',*,*,#9115,.T.);
#13291=ORIENTED_EDGE('',*,*,#9120,.F.);
#13292=ORIENTED_EDGE('',*,*,#9121,.F.);
#13293=ORIENTED_EDGE('',*,*,#9122,.T.);
#13294=ORIENTED_EDGE('',*,*,#9118,.T.);
#13295=ORIENTED_EDGE('',*,*,#9123,.F.);
#13296=ORIENTED_EDGE('',*,*,#9124,.F.);
#13297=ORIENTED_EDGE('',*,*,#9125,.T.);
#13298=ORIENTED_EDGE('',*,*,#9121,.T.);
#13299=ORIENTED_EDGE('',*,*,#9126,.F.);
#13300=ORIENTED_EDGE('',*,*,#9127,.F.);
#13301=ORIENTED_EDGE('',*,*,#9128,.T.);
#13302=ORIENTED_EDGE('',*,*,#9124,.T.);
#13303=ORIENTED_EDGE('',*,*,#9129,.F.);
#13304=ORIENTED_EDGE('',*,*,#9130,.F.);
#13305=ORIENTED_EDGE('',*,*,#9131,.T.);
#13306=ORIENTED_EDGE('',*,*,#9127,.T.);
#13307=ORIENTED_EDGE('',*,*,#9132,.F.);
#13308=ORIENTED_EDGE('',*,*,#9133,.F.);
#13309=ORIENTED_EDGE('',*,*,#9134,.F.);
#13310=ORIENTED_EDGE('',*,*,#9080,.F.);
#13311=ORIENTED_EDGE('',*,*,#9076,.F.);
#13312=ORIENTED_EDGE('',*,*,#9073,.F.);
#13313=ORIENTED_EDGE('',*,*,#9070,.F.);
#13314=ORIENTED_EDGE('',*,*,#9067,.F.);
#13315=ORIENTED_EDGE('',*,*,#9064,.F.);
#13316=ORIENTED_EDGE('',*,*,#9061,.F.);
#13317=ORIENTED_EDGE('',*,*,#9058,.F.);
#13318=ORIENTED_EDGE('',*,*,#9055,.F.);
#13319=ORIENTED_EDGE('',*,*,#9052,.F.);
#13320=ORIENTED_EDGE('',*,*,#9049,.F.);
#13321=ORIENTED_EDGE('',*,*,#9046,.F.);
#13322=ORIENTED_EDGE('',*,*,#9043,.F.);
#13323=ORIENTED_EDGE('',*,*,#9040,.F.);
#13324=ORIENTED_EDGE('',*,*,#9037,.F.);
#13325=ORIENTED_EDGE('',*,*,#9034,.F.);
#13326=ORIENTED_EDGE('',*,*,#9031,.F.);
#13327=ORIENTED_EDGE('',*,*,#9028,.F.);
#13328=ORIENTED_EDGE('',*,*,#9135,.F.);
#13329=ORIENTED_EDGE('',*,*,#9136,.T.);
#13330=ORIENTED_EDGE('',*,*,#9132,.T.);
#13331=ORIENTED_EDGE('',*,*,#9129,.T.);
#13332=ORIENTED_EDGE('',*,*,#9126,.T.);
#13333=ORIENTED_EDGE('',*,*,#9123,.T.);
#13334=ORIENTED_EDGE('',*,*,#9120,.T.);
#13335=ORIENTED_EDGE('',*,*,#9117,.T.);
#13336=ORIENTED_EDGE('',*,*,#9114,.T.);
#13337=ORIENTED_EDGE('',*,*,#9111,.T.);
#13338=ORIENTED_EDGE('',*,*,#9108,.T.);
#13339=ORIENTED_EDGE('',*,*,#9105,.T.);
#13340=ORIENTED_EDGE('',*,*,#9102,.T.);
#13341=ORIENTED_EDGE('',*,*,#9099,.T.);
#13342=ORIENTED_EDGE('',*,*,#9096,.T.);
#13343=ORIENTED_EDGE('',*,*,#9093,.T.);
#13344=ORIENTED_EDGE('',*,*,#9090,.T.);
#13345=ORIENTED_EDGE('',*,*,#9087,.T.);
#13346=ORIENTED_EDGE('',*,*,#9084,.T.);
#13347=ORIENTED_EDGE('',*,*,#9137,.T.);
#13348=ORIENTED_EDGE('',*,*,#9138,.T.);
#13349=ORIENTED_EDGE('',*,*,#9139,.T.);
#13350=ORIENTED_EDGE('',*,*,#9140,.T.);
#13351=ORIENTED_EDGE('',*,*,#9135,.T.);
#13352=ORIENTED_EDGE('',*,*,#9130,.T.);
#13353=ORIENTED_EDGE('',*,*,#9136,.F.);
#13354=ORIENTED_EDGE('',*,*,#9140,.F.);
#13355=ORIENTED_EDGE('',*,*,#9141,.T.);
#13356=ORIENTED_EDGE('',*,*,#9142,.F.);
#13357=ORIENTED_EDGE('',*,*,#9082,.F.);
#13358=ORIENTED_EDGE('',*,*,#9086,.F.);
#13359=ORIENTED_EDGE('',*,*,#9089,.F.);
#13360=ORIENTED_EDGE('',*,*,#9092,.F.);
#13361=ORIENTED_EDGE('',*,*,#9095,.F.);
#13362=ORIENTED_EDGE('',*,*,#9098,.F.);
#13363=ORIENTED_EDGE('',*,*,#9101,.F.);
#13364=ORIENTED_EDGE('',*,*,#9104,.F.);
#13365=ORIENTED_EDGE('',*,*,#9107,.F.);
#13366=ORIENTED_EDGE('',*,*,#9110,.F.);
#13367=ORIENTED_EDGE('',*,*,#9113,.F.);
#13368=ORIENTED_EDGE('',*,*,#9116,.F.);
#13369=ORIENTED_EDGE('',*,*,#9119,.F.);
#13370=ORIENTED_EDGE('',*,*,#9122,.F.);
#13371=ORIENTED_EDGE('',*,*,#9125,.F.);
#13372=ORIENTED_EDGE('',*,*,#9128,.F.);
#13373=ORIENTED_EDGE('',*,*,#9131,.F.);
#13374=ORIENTED_EDGE('',*,*,#9141,.F.);
#13375=ORIENTED_EDGE('',*,*,#9139,.F.);
#13376=ORIENTED_EDGE('',*,*,#9026,.F.);
#13377=ORIENTED_EDGE('',*,*,#9030,.F.);
#13378=ORIENTED_EDGE('',*,*,#9033,.F.);
#13379=ORIENTED_EDGE('',*,*,#9036,.F.);
#13380=ORIENTED_EDGE('',*,*,#9039,.F.);
#13381=ORIENTED_EDGE('',*,*,#9042,.F.);
#13382=ORIENTED_EDGE('',*,*,#9045,.F.);
#13383=ORIENTED_EDGE('',*,*,#9048,.F.);
#13384=ORIENTED_EDGE('',*,*,#9051,.F.);
#13385=ORIENTED_EDGE('',*,*,#9054,.F.);
#13386=ORIENTED_EDGE('',*,*,#9057,.F.);
#13387=ORIENTED_EDGE('',*,*,#9060,.F.);
#13388=ORIENTED_EDGE('',*,*,#9063,.F.);
#13389=ORIENTED_EDGE('',*,*,#9066,.F.);
#13390=ORIENTED_EDGE('',*,*,#9069,.F.);
#13391=ORIENTED_EDGE('',*,*,#9072,.F.);
#13392=ORIENTED_EDGE('',*,*,#9075,.F.);
#13393=ORIENTED_EDGE('',*,*,#9079,.F.);
#13394=ORIENTED_EDGE('',*,*,#9143,.T.);
#13395=ORIENTED_EDGE('',*,*,#9144,.F.);
#13396=ORIENTED_EDGE('',*,*,#9143,.F.);
#13397=ORIENTED_EDGE('',*,*,#9145,.F.);
#13398=ORIENTED_EDGE('',*,*,#9146,.T.);
#13399=ORIENTED_EDGE('',*,*,#9147,.T.);
#13400=ORIENTED_EDGE('',*,*,#9148,.F.);
#13401=ORIENTED_EDGE('',*,*,#9149,.F.);
#13402=ORIENTED_EDGE('',*,*,#9148,.T.);
#13403=ORIENTED_EDGE('',*,*,#9150,.T.);
#13404=ORIENTED_EDGE('',*,*,#9151,.F.);
#13405=ORIENTED_EDGE('',*,*,#9152,.F.);
#13406=ORIENTED_EDGE('',*,*,#9151,.T.);
#13407=ORIENTED_EDGE('',*,*,#9153,.T.);
#13408=ORIENTED_EDGE('',*,*,#9154,.F.);
#13409=ORIENTED_EDGE('',*,*,#9155,.F.);
#13410=ORIENTED_EDGE('',*,*,#9154,.T.);
#13411=ORIENTED_EDGE('',*,*,#9156,.T.);
#13412=ORIENTED_EDGE('',*,*,#9157,.F.);
#13413=ORIENTED_EDGE('',*,*,#9158,.F.);
#13414=ORIENTED_EDGE('',*,*,#9159,.T.);
#13415=ORIENTED_EDGE('',*,*,#9160,.T.);
#13416=ORIENTED_EDGE('',*,*,#9146,.F.);
#13417=ORIENTED_EDGE('',*,*,#9161,.F.);
#13418=ORIENTED_EDGE('',*,*,#9157,.T.);
#13419=ORIENTED_EDGE('',*,*,#9162,.T.);
#13420=ORIENTED_EDGE('',*,*,#9159,.F.);
#13421=ORIENTED_EDGE('',*,*,#9162,.F.);
#13422=ORIENTED_EDGE('',*,*,#9156,.F.);
#13423=ORIENTED_EDGE('',*,*,#9153,.F.);
#13424=ORIENTED_EDGE('',*,*,#9150,.F.);
#13425=ORIENTED_EDGE('',*,*,#9147,.F.);
#13426=ORIENTED_EDGE('',*,*,#9160,.F.);
#13427=ORIENTED_EDGE('',*,*,#9144,.T.);
#13428=ORIENTED_EDGE('',*,*,#9163,.F.);
#13429=ORIENTED_EDGE('',*,*,#9137,.F.);
#13430=ORIENTED_EDGE('',*,*,#9027,.F.);
#13431=ORIENTED_EDGE('',*,*,#9138,.F.);
#13432=ORIENTED_EDGE('',*,*,#9164,.T.);
#13433=ORIENTED_EDGE('',*,*,#9163,.T.);
#13434=ORIENTED_EDGE('',*,*,#9164,.F.);
#13435=ORIENTED_EDGE('',*,*,#9077,.T.);
#13436=ORIENTED_EDGE('',*,*,#9134,.T.);
#13437=ORIENTED_EDGE('',*,*,#9165,.F.);
#13438=ORIENTED_EDGE('',*,*,#9166,.F.);
#13439=ORIENTED_EDGE('',*,*,#9078,.T.);
#13440=ORIENTED_EDGE('',*,*,#9165,.T.);
#13441=ORIENTED_EDGE('',*,*,#9133,.T.);
#13442=ORIENTED_EDGE('',*,*,#9083,.T.);
#13443=ORIENTED_EDGE('',*,*,#9142,.T.);
#13444=ORIENTED_EDGE('',*,*,#9167,.F.);
#13445=ORIENTED_EDGE('',*,*,#9168,.T.);
#13446=ORIENTED_EDGE('',*,*,#9166,.T.);
#13447=ORIENTED_EDGE('',*,*,#9168,.F.);
#13448=ORIENTED_EDGE('',*,*,#9169,.F.);
#13449=ORIENTED_EDGE('',*,*,#9155,.T.);
#13450=ORIENTED_EDGE('',*,*,#9161,.T.);
#13451=ORIENTED_EDGE('',*,*,#9158,.T.);
#13452=ORIENTED_EDGE('',*,*,#9145,.T.);
#13453=ORIENTED_EDGE('',*,*,#9149,.T.);
#13454=ORIENTED_EDGE('',*,*,#9152,.T.);
#13455=ORIENTED_EDGE('',*,*,#9170,.T.);
#13456=ORIENTED_EDGE('',*,*,#9169,.T.);
#13457=ORIENTED_EDGE('',*,*,#9167,.T.);
#13458=ORIENTED_EDGE('',*,*,#9170,.F.);
#13926=PLANE('',#16078);
#13927=PLANE('',#16085);
#13928=PLANE('',#16086);
#13929=PLANE('',#16087);
#13930=PLANE('',#16088);
#13931=PLANE('',#16089);
#13932=PLANE('',#16090);
#13933=PLANE('',#16091);
#13934=PLANE('',#16092);
#13935=PLANE('',#16097);
#14723=ADVANCED_FACE('',(#2155),#913,.T.);
#14724=ADVANCED_FACE('',(#2156),#914,.T.);
#14725=ADVANCED_FACE('',(#2157),#915,.T.);
#14726=ADVANCED_FACE('',(#2158),#916,.T.);
#14727=ADVANCED_FACE('',(#2159),#917,.T.);
#14728=ADVANCED_FACE('',(#2160),#918,.T.);
#14729=ADVANCED_FACE('',(#2161),#919,.T.);
#14730=ADVANCED_FACE('',(#2162),#920,.T.);
#14731=ADVANCED_FACE('',(#2163),#921,.T.);
#14732=ADVANCED_FACE('',(#2164),#922,.T.);
#14733=ADVANCED_FACE('',(#2165),#923,.T.);
#14734=ADVANCED_FACE('',(#2166),#924,.T.);
#14735=ADVANCED_FACE('',(#2167),#925,.T.);
#14736=ADVANCED_FACE('',(#2168),#926,.T.);
#14737=ADVANCED_FACE('',(#2169),#927,.T.);
#14738=ADVANCED_FACE('',(#2170),#928,.T.);
#14739=ADVANCED_FACE('',(#2171),#929,.T.);
#14740=ADVANCED_FACE('',(#2172),#930,.T.);
#14741=ADVANCED_FACE('',(#2173),#931,.T.);
#14742=ADVANCED_FACE('',(#2174),#932,.T.);
#14743=ADVANCED_FACE('',(#2175),#933,.T.);
#14744=ADVANCED_FACE('',(#2176),#934,.T.);
#14745=ADVANCED_FACE('',(#2177),#935,.T.);
#14746=ADVANCED_FACE('',(#2178),#936,.T.);
#14747=ADVANCED_FACE('',(#2179),#937,.T.);
#14748=ADVANCED_FACE('',(#2180),#938,.T.);
#14749=ADVANCED_FACE('',(#2181),#939,.T.);
#14750=ADVANCED_FACE('',(#2182),#940,.T.);
#14751=ADVANCED_FACE('',(#2183),#941,.T.);
#14752=ADVANCED_FACE('',(#2184),#942,.T.);
#14753=ADVANCED_FACE('',(#2185),#943,.T.);
#14754=ADVANCED_FACE('',(#2186),#944,.T.);
#14755=ADVANCED_FACE('',(#2187),#945,.T.);
#14756=ADVANCED_FACE('',(#2188),#946,.T.);
#14757=ADVANCED_FACE('',(#2189),#947,.T.);
#14758=ADVANCED_FACE('',(#2190),#118,.F.);
#14759=ADVANCED_FACE('',(#2191),#13926,.T.);
#14760=ADVANCED_FACE('',(#2192),#948,.T.);
#14761=ADVANCED_FACE('',(#2193),#119,.F.);
#14762=ADVANCED_FACE('',(#2194),#1366,.F.);
#14763=ADVANCED_FACE('',(#2195),#13927,.F.);
#14764=ADVANCED_FACE('',(#2196),#13928,.F.);
#14765=ADVANCED_FACE('',(#2197),#13929,.F.);
#14766=ADVANCED_FACE('',(#2198),#13930,.F.);
#14767=ADVANCED_FACE('',(#2199),#13931,.F.);
#14768=ADVANCED_FACE('',(#2200),#13932,.F.);
#14769=ADVANCED_FACE('',(#2201,#688),#13933,.F.);
#14770=ADVANCED_FACE('',(#2202),#13934,.T.);
#14771=ADVANCED_FACE('',(#2203),#1367,.T.);
#14772=ADVANCED_FACE('',(#2204),#949,.T.);
#14773=ADVANCED_FACE('',(#2205,#689),#13935,.T.);
#14774=ADVANCED_FACE('',(#2206),#950,.T.);
#14775=ADVANCED_FACE('',(#2207),#104,.F.);
#14788=CLOSED_SHELL('',(#14723,#14724,#14725,#14726,#14727,#14728,#14729,
#14730,#14731,#14732,#14733,#14734,#14735,#14736,#14737,#14738,#14739,#14740,
#14741,#14742,#14743,#14744,#14745,#14746,#14747,#14748,#14749,#14750,#14751,
#14752,#14753,#14754,#14755,#14756,#14757,#14758,#14759,#14760,#14761,#14762,
#14763,#14764,#14765,#14766,#14767,#14768,#14769,#14770,#14771,#14772,#14773,
#14774,#14775));
#16039=AXIS2_PLACEMENT_3D('',#34457,#19526,#19527);
#16040=AXIS2_PLACEMENT_3D('',#34458,#19528,#19529);
#16041=AXIS2_PLACEMENT_3D('',#34474,#19531,#19532);
#16042=AXIS2_PLACEMENT_3D('',#34482,#19533,#19534);
#16043=AXIS2_PLACEMENT_3D('',#34530,#19536,#19537);
#16044=AXIS2_PLACEMENT_3D('',#34578,#19539,#19540);
#16045=AXIS2_PLACEMENT_3D('',#34629,#19542,#19543);
#16046=AXIS2_PLACEMENT_3D('',#34680,#19545,#19546);
#16047=AXIS2_PLACEMENT_3D('',#34728,#19548,#19549);
#16048=AXIS2_PLACEMENT_3D('',#34776,#19551,#19552);
#16049=AXIS2_PLACEMENT_3D('',#34830,#19554,#19555);
#16050=AXIS2_PLACEMENT_3D('',#34878,#19557,#19558);
#16051=AXIS2_PLACEMENT_3D('',#34926,#19560,#19561);
#16052=AXIS2_PLACEMENT_3D('',#34980,#19563,#19564);
#16053=AXIS2_PLACEMENT_3D('',#35028,#19566,#19567);
#16054=AXIS2_PLACEMENT_3D('',#35076,#19569,#19570);
#16055=AXIS2_PLACEMENT_3D('',#35124,#19572,#19573);
#16056=AXIS2_PLACEMENT_3D('',#35178,#19575,#19576);
#16057=AXIS2_PLACEMENT_3D('',#35226,#19578,#19579);
#16058=AXIS2_PLACEMENT_3D('',#35274,#19581,#19582);
#16059=AXIS2_PLACEMENT_3D('',#35279,#19584,#19585);
#16060=AXIS2_PLACEMENT_3D('',#35327,#19586,#19587);
#16061=AXIS2_PLACEMENT_3D('',#35341,#19589,#19590);
#16062=AXIS2_PLACEMENT_3D('',#35348,#19591,#19592);
#16063=AXIS2_PLACEMENT_3D('',#35373,#19594,#19595);
#16064=AXIS2_PLACEMENT_3D('',#35397,#19597,#19598);
#16065=AXIS2_PLACEMENT_3D('',#35422,#19600,#19601);
#16066=AXIS2_PLACEMENT_3D('',#35447,#19603,#19604);
#16067=AXIS2_PLACEMENT_3D('',#35471,#19606,#19607);
#16068=AXIS2_PLACEMENT_3D('',#35495,#19609,#19610);
#16069=AXIS2_PLACEMENT_3D('',#35520,#19612,#19613);
#16070=AXIS2_PLACEMENT_3D('',#35545,#19615,#19616);
#16071=AXIS2_PLACEMENT_3D('',#35569,#19618,#19619);
#16072=AXIS2_PLACEMENT_3D('',#35594,#19621,#19622);
#16073=AXIS2_PLACEMENT_3D('',#35619,#19624,#19625);
#16074=AXIS2_PLACEMENT_3D('',#35643,#19627,#19628);
#16075=AXIS2_PLACEMENT_3D('',#35668,#19630,#19631);
#16076=AXIS2_PLACEMENT_3D('',#35692,#19633,#19634);
#16077=AXIS2_PLACEMENT_3D('',#35717,#19636,#19637);
#16078=AXIS2_PLACEMENT_3D('',#36376,#19639,#19640);
#16079=AXIS2_PLACEMENT_3D('',#36378,#19641,#19642);
#16080=AXIS2_PLACEMENT_3D('',#36379,#19643,#19644);
#16081=AXIS2_PLACEMENT_3D('',#36463,#19645,#19646);
#16082=AXIS2_PLACEMENT_3D('',#36464,#19647,#19648);
#16083=AXIS2_PLACEMENT_3D('',#37011,#19649,#19650);
#16084=AXIS2_PLACEMENT_3D('',#37015,#19652,#19653);
#16085=AXIS2_PLACEMENT_3D('',#37016,#19654,#19655);
#16086=AXIS2_PLACEMENT_3D('',#37030,#19659,#19660);
#16087=AXIS2_PLACEMENT_3D('',#37041,#19663,#19664);
#16088=AXIS2_PLACEMENT_3D('',#37052,#19667,#19668);
#16089=AXIS2_PLACEMENT_3D('',#37063,#19671,#19672);
#16090=AXIS2_PLACEMENT_3D('',#37074,#19675,#19676);
#16091=AXIS2_PLACEMENT_3D('',#37082,#19678,#19679);
#16092=AXIS2_PLACEMENT_3D('',#37083,#19680,#19681);
#16093=AXIS2_PLACEMENT_3D('',#37085,#19682,#19683);
#16094=AXIS2_PLACEMENT_3D('',#37086,#19684,#19685);
#16095=AXIS2_PLACEMENT_3D('',#37088,#19687,#19688);
#16096=AXIS2_PLACEMENT_3D('',#37089,#19689,#19690);
#16097=AXIS2_PLACEMENT_3D('',#37090,#19691,#19692);
#16098=AXIS2_PLACEMENT_3D('',#37092,#19693,#19694);
#16099=AXIS2_PLACEMENT_3D('',#37093,#19695,#19696);
#16100=AXIS2_PLACEMENT_3D('',#37096,#19697,#19698);
#16101=AXIS2_PLACEMENT_3D('',#37098,#19700,#19701);
#19526=DIRECTION('axis',(0.,0.,1.));
#19527=DIRECTION('refdir',(1.,0.,0.));
#19528=DIRECTION('center_axis',(1.,0.,0.));
#19529=DIRECTION('ref_axis',(0.,1.,0.));
#19530=DIRECTION('',(-1.,0.,0.));
#19531=DIRECTION('center_axis',(1.,0.,0.));
#19532=DIRECTION('ref_axis',(0.,1.,0.));
#19533=DIRECTION('center_axis',(1.,0.,0.));
#19534=DIRECTION('ref_axis',(0.,1.,0.));
#19535=DIRECTION('',(-1.,0.,0.));
#19536=DIRECTION('center_axis',(1.,0.,0.));
#19537=DIRECTION('ref_axis',(0.,1.,0.));
#19538=DIRECTION('',(-1.,0.,0.));
#19539=DIRECTION('center_axis',(1.,0.,0.));
#19540=DIRECTION('ref_axis',(0.,1.,0.));
#19541=DIRECTION('',(-1.,0.,0.));
#19542=DIRECTION('center_axis',(1.,0.,0.));
#19543=DIRECTION('ref_axis',(0.,1.,0.));
#19544=DIRECTION('',(-1.,0.,0.));
#19545=DIRECTION('center_axis',(1.,0.,0.));
#19546=DIRECTION('ref_axis',(0.,1.,0.));
#19547=DIRECTION('',(-1.,0.,0.));
#19548=DIRECTION('center_axis',(1.,0.,0.));
#19549=DIRECTION('ref_axis',(0.,1.,0.));
#19550=DIRECTION('',(-1.,0.,0.));
#19551=DIRECTION('center_axis',(1.,0.,0.));
#19552=DIRECTION('ref_axis',(0.,1.,0.));
#19553=DIRECTION('',(-1.,0.,0.));
#19554=DIRECTION('center_axis',(1.,0.,0.));
#19555=DIRECTION('ref_axis',(0.,1.,0.));
#19556=DIRECTION('',(-1.,0.,0.));
#19557=DIRECTION('center_axis',(1.,0.,0.));
#19558=DIRECTION('ref_axis',(0.,1.,0.));
#19559=DIRECTION('',(-1.,0.,0.));
#19560=DIRECTION('center_axis',(1.,0.,0.));
#19561=DIRECTION('ref_axis',(0.,1.,0.));
#19562=DIRECTION('',(-1.,0.,0.));
#19563=DIRECTION('center_axis',(1.,0.,0.));
#19564=DIRECTION('ref_axis',(0.,1.,0.));
#19565=DIRECTION('',(-1.,0.,0.));
#19566=DIRECTION('center_axis',(1.,0.,0.));
#19567=DIRECTION('ref_axis',(0.,1.,0.));
#19568=DIRECTION('',(-1.,0.,0.));
#19569=DIRECTION('center_axis',(1.,0.,0.));
#19570=DIRECTION('ref_axis',(0.,1.,0.));
#19571=DIRECTION('',(-1.,0.,0.));
#19572=DIRECTION('center_axis',(1.,0.,0.));
#19573=DIRECTION('ref_axis',(0.,1.,0.));
#19574=DIRECTION('',(-1.,0.,0.));
#19575=DIRECTION('center_axis',(1.,0.,0.));
#19576=DIRECTION('ref_axis',(0.,1.,0.));
#19577=DIRECTION('',(-1.,0.,0.));
#19578=DIRECTION('center_axis',(1.,0.,0.));
#19579=DIRECTION('ref_axis',(0.,1.,0.));
#19580=DIRECTION('',(-1.,0.,0.));
#19581=DIRECTION('center_axis',(1.,0.,0.));
#19582=DIRECTION('ref_axis',(0.,1.,0.));
#19583=DIRECTION('',(-1.,0.,0.));
#19584=DIRECTION('center_axis',(1.,0.,0.));
#19585=DIRECTION('ref_axis',(0.,1.,0.));
#19586=DIRECTION('center_axis',(1.,0.,0.));
#19587=DIRECTION('ref_axis',(0.,0.449886232649206,-0.893085873627337));
#19588=DIRECTION('',(1.,0.,0.));
#19589=DIRECTION('center_axis',(1.,0.,0.));
#19590=DIRECTION('ref_axis',(0.,1.,1.377013058433E-13));
#19591=DIRECTION('center_axis',(1.,0.,0.));
#19592=DIRECTION('ref_axis',(0.,1.,1.377013058433E-13));
#19593=DIRECTION('',(1.,0.,0.));
#19594=DIRECTION('center_axis',(1.,0.,0.));
#19595=DIRECTION('ref_axis',(0.,1.,1.377013058433E-13));
#19596=DIRECTION('',(1.,0.,0.));
#19597=DIRECTION('center_axis',(1.,0.,0.));
#19598=DIRECTION('ref_axis',(0.,1.,1.377013058433E-13));
#19599=DIRECTION('',(1.,0.,0.));
#19600=DIRECTION('center_axis',(1.,0.,0.));
#19601=DIRECTION('ref_axis',(0.,1.,1.377013058433E-13));
#19602=DIRECTION('',(1.,0.,0.));
#19603=DIRECTION('center_axis',(1.,0.,0.));
#19604=DIRECTION('ref_axis',(0.,1.,1.377013058433E-13));
#19605=DIRECTION('',(1.,0.,0.));
#19606=DIRECTION('center_axis',(1.,0.,0.));
#19607=DIRECTION('ref_axis',(0.,1.,1.377013058433E-13));
#19608=DIRECTION('',(1.,0.,0.));
#19609=DIRECTION('center_axis',(1.,0.,0.));
#19610=DIRECTION('ref_axis',(0.,1.,1.377013058433E-13));
#19611=DIRECTION('',(1.,0.,0.));
#19612=DIRECTION('center_axis',(1.,0.,0.));
#19613=DIRECTION('ref_axis',(0.,1.,1.377013058433E-13));
#19614=DIRECTION('',(1.,0.,0.));
#19615=DIRECTION('center_axis',(1.,0.,0.));
#19616=DIRECTION('ref_axis',(0.,1.,1.377013058433E-13));
#19617=DIRECTION('',(1.,0.,0.));
#19618=DIRECTION('center_axis',(1.,0.,0.));
#19619=DIRECTION('ref_axis',(0.,1.,1.377013058433E-13));
#19620=DIRECTION('',(1.,0.,0.));
#19621=DIRECTION('center_axis',(1.,0.,0.));
#19622=DIRECTION('ref_axis',(0.,1.,1.377013058433E-13));
#19623=DIRECTION('',(1.,0.,0.));
#19624=DIRECTION('center_axis',(1.,0.,0.));
#19625=DIRECTION('ref_axis',(0.,1.,1.377013058433E-13));
#19626=DIRECTION('',(1.,0.,0.));
#19627=DIRECTION('center_axis',(1.,0.,0.));
#19628=DIRECTION('ref_axis',(0.,1.,1.377013058433E-13));
#19629=DIRECTION('',(1.,0.,0.));
#19630=DIRECTION('center_axis',(1.,0.,0.));
#19631=DIRECTION('ref_axis',(0.,1.,1.377013058433E-13));
#19632=DIRECTION('',(1.,0.,0.));
#19633=DIRECTION('center_axis',(1.,0.,0.));
#19634=DIRECTION('ref_axis',(0.,1.,1.377013058433E-13));
#19635=DIRECTION('',(1.,0.,0.));
#19636=DIRECTION('center_axis',(1.,0.,0.));
#19637=DIRECTION('ref_axis',(0.,1.,1.377013058433E-13));
#19638=DIRECTION('',(1.,0.,0.));
#19639=DIRECTION('center_axis',(1.,0.,0.));
#19640=DIRECTION('ref_axis',(0.,0.,-1.));
#19641=DIRECTION('center_axis',(1.,0.,0.));
#19642=DIRECTION('ref_axis',(0.,1.,0.));
#19643=DIRECTION('center_axis',(1.,0.,0.));
#19644=DIRECTION('ref_axis',(0.,1.,0.));
#19645=DIRECTION('center_axis',(-1.,0.,0.));
#19646=DIRECTION('ref_axis',(0.,1.,1.377013058433E-13));
#19647=DIRECTION('center_axis',(1.,0.,0.));
#19648=DIRECTION('ref_axis',(0.,1.,1.377013058433E-13));
#19649=DIRECTION('center_axis',(1.,0.,0.));
#19650=DIRECTION('ref_axis',(0.,1.,0.));
#19651=DIRECTION('',(0.523361335187425,-0.852110857125313,-1.04353483369722E-16));
#19652=DIRECTION('center_axis',(-1.,0.,0.));
#19653=DIRECTION('ref_axis',(0.,1.,0.));
#19654=DIRECTION('center_axis',(0.,-0.5,-0.866025403784439));
#19655=DIRECTION('ref_axis',(0.,-0.866025403784439,0.5));
#19656=DIRECTION('',(-1.,0.,0.));
#19657=DIRECTION('',(0.,-0.866025403784439,0.5));
#19658=DIRECTION('',(-1.,0.,0.));
#19659=DIRECTION('center_axis',(0.,-1.,-1.60246890531964E-16));
#19660=DIRECTION('ref_axis',(0.,-1.60246890531964E-16,1.));
#19661=DIRECTION('',(0.,-1.60246890531964E-16,1.));
#19662=DIRECTION('',(-1.,0.,0.));
#19663=DIRECTION('center_axis',(0.,-0.5,0.866025403784439));
#19664=DIRECTION('ref_axis',(0.,0.866025403784439,0.5));
#19665=DIRECTION('',(0.,0.866025403784439,0.5));
#19666=DIRECTION('',(-1.,0.,0.));
#19667=DIRECTION('center_axis',(0.,0.5,0.866025403784439));
#19668=DIRECTION('ref_axis',(0.,0.866025403784439,-0.5));
#19669=DIRECTION('',(0.,0.866025403784439,-0.5));
#19670=DIRECTION('',(-1.,0.,0.));
#19671=DIRECTION('center_axis',(0.,0.5,-0.866025403784439));
#19672=DIRECTION('ref_axis',(0.,-0.866025403784439,-0.5));
#19673=DIRECTION('',(-1.,0.,0.));
#19674=DIRECTION('',(0.,-0.866025403784439,-0.5));
#19675=DIRECTION('center_axis',(0.,1.,-3.20493781063927E-16));
#19676=DIRECTION('ref_axis',(0.,-3.20493781063927E-16,-1.));
#19677=DIRECTION('',(0.,-3.20493781063927E-16,-1.));
#19678=DIRECTION('center_axis',(-1.,0.,0.));
#19679=DIRECTION('ref_axis',(0.,0.,1.));
#19680=DIRECTION('center_axis',(-1.,0.,0.));
#19681=DIRECTION('ref_axis',(0.,0.,1.));
#19682=DIRECTION('center_axis',(1.,0.,0.));
#19683=DIRECTION('ref_axis',(0.,0.,-1.));
#19684=DIRECTION('center_axis',(1.,0.,0.));
#19685=DIRECTION('ref_axis',(0.,1.,0.));
#19686=DIRECTION('',(-0.707106781186548,0.707106781186547,8.65956056235493E-17));
#19687=DIRECTION('center_axis',(1.,0.,0.));
#19688=DIRECTION('ref_axis',(0.,-0.927547100086637,-0.373706271182154));
#19689=DIRECTION('center_axis',(1.,0.,0.));
#19690=DIRECTION('ref_axis',(0.,1.,0.));
#19691=DIRECTION('center_axis',(-1.,0.,0.));
#19692=DIRECTION('ref_axis',(0.,0.,1.));
#19693=DIRECTION('center_axis',(1.,0.,0.));
#19694=DIRECTION('ref_axis',(0.,0.,-1.));
#19695=DIRECTION('center_axis',(1.,0.,0.));
#19696=DIRECTION('ref_axis',(0.,1.,0.));
#19697=DIRECTION('center_axis',(1.,0.,0.));
#19698=DIRECTION('ref_axis',(0.,0.,-1.));
#19699=DIRECTION('',(-1.,0.,0.));
#19700=DIRECTION('center_axis',(1.,0.,0.));
#19701=DIRECTION('ref_axis',(0.,0.,-1.));
#34457=CARTESIAN_POINT('',(0.,0.,0.));
#34458=CARTESIAN_POINT('Origin',(-3.875,0.,0.));
#34459=CARTESIAN_POINT('',(-7.64010734985006,-1.21647452716103,0.000783377930972141));
#34460=CARTESIAN_POINT('',(-7.70489265014995,-1.21612319654208,0.00132237507692805));
#34461=CARTESIAN_POINT('',(-3.875,-1.215,-1.48794586096403E-16));
#34462=CARTESIAN_POINT('',(-7.785,0.531620960029506,1.09362937143029));
#34463=CARTESIAN_POINT('Ctrl Pts',(-7.64010734985006,-1.21647452716103,
0.000783377930972141));
#34464=CARTESIAN_POINT('Ctrl Pts',(-7.64252235014853,-1.21675455720845,
0.0416081919322704));
#34465=CARTESIAN_POINT('Ctrl Pts',(-7.64493735044699,-1.21487817361819,
0.0824052162368853));
#34466=CARTESIAN_POINT('Ctrl Pts',(-7.64735235074546,-1.21076076162991,
0.122972630877474));
#34467=CARTESIAN_POINT('Ctrl Pts',(-7.67117587831787,-1.17014326021919,
0.523162610914586));
#34468=CARTESIAN_POINT('Ctrl Pts',(-7.69499940589029,-0.911441098580177,
0.901008230831576));
#34469=CARTESIAN_POINT('Ctrl Pts',(-7.7188229334627,-0.553047883833515,
1.08394887030055));
#34470=CARTESIAN_POINT('Ctrl Pts',(-7.7408819556418,-0.221199300582993,
1.25333988979749));
#34471=CARTESIAN_POINT('Ctrl Pts',(-7.7629409778209,0.196119845112543,1.25562826785441));
#34472=CARTESIAN_POINT('Ctrl Pts',(-7.785,0.532258410758873,1.09442686519078));
#34473=CARTESIAN_POINT('',(-7.785,-0.530983509300163,1.09283187766979));
#34474=CARTESIAN_POINT('Origin',(-7.785,0.,0.));
#34475=CARTESIAN_POINT('Ctrl Pts',(-7.785,-0.530983509300162,1.09283187766979));
#34476=CARTESIAN_POINT('Ctrl Pts',(-7.76117647242759,-0.894502226956994,
0.916205949801275));
#34477=CARTESIAN_POINT('Ctrl Pts',(-7.73735294485517,-1.15982398095655,
0.54548974214433));
#34478=CARTESIAN_POINT('Ctrl Pts',(-7.71352941728276,-1.20802527945981,
0.146755193366327));
#34479=CARTESIAN_POINT('Ctrl Pts',(-7.71065049490516,-1.21385010101357,
0.0985706492550221));
#34480=CARTESIAN_POINT('Ctrl Pts',(-7.70777157252755,-1.21650427102171,
0.0499769479485646));
#34481=CARTESIAN_POINT('Ctrl Pts',(-7.70489265014995,-1.21612319654208,
0.00132237507692805));
#34482=CARTESIAN_POINT('Origin',(-3.875,0.,0.));
#34483=CARTESIAN_POINT('',(-7.19010734985006,-1.21334095132918,0.000643174960512083));
#34484=CARTESIAN_POINT('',(-7.25489265014995,-1.21322307873259,0.000540336490138318));
#34485=CARTESIAN_POINT('',(-3.875,-1.215,-1.48794586096403E-16));
#34486=CARTESIAN_POINT('Ctrl Pts',(-7.19010734985006,-1.21334095132918,
0.000643174960512083));
#34487=CARTESIAN_POINT('Ctrl Pts',(-7.19958118471403,-1.21411261089513,
0.161870787822646));
#34488=CARTESIAN_POINT('Ctrl Pts',(-7.209055019578,-1.18425339306602,0.322823852770454));
#34489=CARTESIAN_POINT('Ctrl Pts',(-7.21852885444197,-1.12241826653371,
0.470375966826099));
#34490=CARTESIAN_POINT('Ctrl Pts',(-7.24235238201438,-0.966923594836523,
0.841420206887963));
#34491=CARTESIAN_POINT('Ctrl Pts',(-7.2661759095868,-0.609227870983272,
1.127722949986));
#34492=CARTESIAN_POINT('Ctrl Pts',(-7.28999943715921,-0.213134957863081,
1.19818283107809));
#34493=CARTESIAN_POINT('Ctrl Pts',(-7.31382296473163,0.182957955257111,
1.26864271217017));
#34494=CARTESIAN_POINT('Ctrl Pts',(-7.33764649230405,0.617448057644243,
1.12325973125629));
#34495=CARTESIAN_POINT('Ctrl Pts',(-7.36147001987647,0.89135892310283,0.828592550610321));
#34496=CARTESIAN_POINT('Ctrl Pts',(-7.38529354744888,1.16526978856142,0.533925369964354));
#34497=CARTESIAN_POINT('Ctrl Pts',(-7.40911707502129,1.27860141709146,0.0899739895862994));
#34498=CARTESIAN_POINT('Ctrl Pts',(-7.43294060259371,1.17945999521821,-0.29991955157041));
#34499=CARTESIAN_POINT('Ctrl Pts',(-7.45676413016612,1.08031857334496,-0.689813092727121));
#34500=CARTESIAN_POINT('Ctrl Pts',(-7.48058765773854,0.768704101068424,
-1.02564879466249));
#34501=CARTESIAN_POINT('Ctrl Pts',(-7.50441118531096,0.38730793589725,-1.15370023444288));
#34502=CARTESIAN_POINT('Ctrl Pts',(-7.52823471288338,0.00591177072607862,
-1.28175167422327));
#34503=CARTESIAN_POINT('Ctrl Pts',(-7.55205824045579,-0.445266087339727,
-1.20201885184869));
#34504=CARTESIAN_POINT('Ctrl Pts',(-7.5758817680282,-0.759588595781406,
-0.950885270582782));
#34505=CARTESIAN_POINT('Ctrl Pts',(-7.59729029530215,-1.0420481087287,-0.725209198573965));
#34506=CARTESIAN_POINT('Ctrl Pts',(-7.61869882257611,-1.21399211301332,
-0.361120984795996));
#34507=CARTESIAN_POINT('Ctrl Pts',(-7.64010734985006,-1.21647452716103,
0.000783377930972141));
#34508=CARTESIAN_POINT('Ctrl Pts',(-7.70489265014995,-1.21612319654208,
0.00132237507692805));
#34509=CARTESIAN_POINT('Ctrl Pts',(-7.68394804495514,-1.213350820813,-0.352647161457663));
#34510=CARTESIAN_POINT('Ctrl Pts',(-7.66300343976032,-1.04992940871555,
-0.709838500495367));
#34511=CARTESIAN_POINT('Ctrl Pts',(-7.64205883456551,-0.777998593308031,
-0.936141314006237));
#34512=CARTESIAN_POINT('Ctrl Pts',(-7.61823530699309,-0.468689765646071,
-1.19355038270171));
#34513=CARTESIAN_POINT('Ctrl Pts',(-7.59441177942068,-0.018991267315219,
-1.28161563019358));
#34514=CARTESIAN_POINT('Ctrl Pts',(-7.57058825184826,0.364858107186471,
-1.16089853528955));
#34515=CARTESIAN_POINT('Ctrl Pts',(-7.54676472427585,0.74870748168816,-1.04018144038552));
#34516=CARTESIAN_POINT('Ctrl Pts',(-7.52294119670343,1.06670773236069,-0.710682003085598));
#34517=CARTESIAN_POINT('Ctrl Pts',(-7.49911766913101,1.17338741195235,-0.322840256676906));
#34518=CARTESIAN_POINT('Ctrl Pts',(-7.47529414155859,1.28006709154401,0.0650014897317872));
#34519=CARTESIAN_POINT('Ctrl Pts',(-7.45147061398618,1.1754262000548,0.511185545249247));
#34520=CARTESIAN_POINT('Ctrl Pts',(-7.42764708641377,0.907302988772841,
0.811146645493936));
#34521=CARTESIAN_POINT('Ctrl Pts',(-7.40382355884135,0.639179777490878,
1.11110774573863));
#34522=CARTESIAN_POINT('Ctrl Pts',(-7.38000003126893,0.20757424641616,1.26484589071055));
#34523=CARTESIAN_POINT('Ctrl Pts',(-7.35617650369652,-0.189818330789957,
1.20208175535973));
#34524=CARTESIAN_POINT('Ctrl Pts',(-7.3323529761241,-0.587210907996071,
1.13931762000892));
#34525=CARTESIAN_POINT('Ctrl Pts',(-7.30852944855169,-0.950390531333583,
0.860051204335379));
#34526=CARTESIAN_POINT('Ctrl Pts',(-7.28470592097928,-1.11306298319363,
0.492106025130156));
#34527=CARTESIAN_POINT('Ctrl Pts',(-7.27476816403617,-1.18092024249372,
0.338621208567414));
#34528=CARTESIAN_POINT('Ctrl Pts',(-7.26483040709306,-1.2138880203146,0.169705741544439));
#34529=CARTESIAN_POINT('Ctrl Pts',(-7.25489265014995,-1.21322307873259,
0.000540336490138318));
#34530=CARTESIAN_POINT('Origin',(-3.875,0.,0.));
#34531=CARTESIAN_POINT('',(-6.74010734985006,-1.21414526361761,-0.00102520398183079));
#34532=CARTESIAN_POINT('',(-6.80489265014995,-1.21436027551958,-0.00106957681048473));
#34533=CARTESIAN_POINT('',(-3.875,-1.215,-1.48794586096403E-16));
#34534=CARTESIAN_POINT('Ctrl Pts',(-6.74010734985006,-1.21414526361761,
-0.00102520398183079));
#34535=CARTESIAN_POINT('Ctrl Pts',(-6.75664001927953,-1.21189888768043,
0.279861953419163));
#34536=CARTESIAN_POINT('Ctrl Pts',(-6.77317268870901,-1.11490370551602,
0.562149070738359));
#34537=CARTESIAN_POINT('Ctrl Pts',(-6.78970535813848,-0.936647874117358,
0.777023963888983));
#34538=CARTESIAN_POINT('Ctrl Pts',(-6.8135288857109,-0.679781750205209,
1.08665804708595));
#34539=CARTESIAN_POINT('Ctrl Pts',(-6.83735241328332,-0.254180127287122,
1.25631250433391));
#34540=CARTESIAN_POINT('Ctrl Pts',(-6.86117594085573,0.145254223191172,
1.20829487101183));
#34541=CARTESIAN_POINT('Ctrl Pts',(-6.88499946842815,0.544688573669464,
1.16027723768975));
#34542=CARTESIAN_POINT('Ctrl Pts',(-6.90882299600056,0.917955651707963,
0.894587513797618));
#34543=CARTESIAN_POINT('Ctrl Pts',(-6.93264652357298,1.0941190081907,0.532896993842244));
#34544=CARTESIAN_POINT('Ctrl Pts',(-6.95647005114539,1.27028236467343,0.171206473886867));
#34545=CARTESIAN_POINT('Ctrl Pts',(-6.98029357871781,1.2493419996004,-0.286484842131756));
#34546=CARTESIAN_POINT('Ctrl Pts',(-7.00411710629023,1.04088761013505,-0.630578012028203));
#34547=CARTESIAN_POINT('Ctrl Pts',(-7.02794063386264,0.832433220669708,
-0.97467118192465));
#34548=CARTESIAN_POINT('Ctrl Pts',(-7.05176416143506,0.436464806812055,
-1.20516620569892));
#34549=CARTESIAN_POINT('Ctrl Pts',(-7.07558768900747,0.0343145048386373,
-1.21651013722172));
#34550=CARTESIAN_POINT('Ctrl Pts',(-7.09941121657989,-0.36783579713478,
-1.22785406874451));
#34551=CARTESIAN_POINT('Ctrl Pts',(-7.1232347441523,-0.776167987223963,
-1.02004690801583));
#34552=CARTESIAN_POINT('Ctrl Pts',(-7.14705827172472,-1.00368727249799,
-0.688250459138645));
#34553=CARTESIAN_POINT('Ctrl Pts',(-7.16140796443317,-1.14072960676204,
-0.488398566144665));
#34554=CARTESIAN_POINT('Ctrl Pts',(-7.17575765714162,-1.21217214505317,
-0.243562760007505));
#34555=CARTESIAN_POINT('Ctrl Pts',(-7.19010734985006,-1.21334095132918,
0.000643174960512083));
#34556=CARTESIAN_POINT('Ctrl Pts',(-7.25489265014995,-1.21322307873259,
0.000540336490138318));
#34557=CARTESIAN_POINT('Ctrl Pts',(-7.24100687952064,-1.21229397306592,
-0.235830106704008));
#34558=CARTESIAN_POINT('Ctrl Pts',(-7.22712110889133,-1.14570118758852,
-0.472688522656612));
#34559=CARTESIAN_POINT('Ctrl Pts',(-7.21323533826202,-1.01687317306236,
-0.668621881745882));
#34560=CARTESIAN_POINT('Ctrl Pts',(-7.18941181068961,-0.795845630688474,
-1.0047806666798));
#34561=CARTESIAN_POINT('Ctrl Pts',(-7.1655882831172,-0.391625265558127,
-1.22047429381071));
#34562=CARTESIAN_POINT('Ctrl Pts',(-7.14176475554478,0.0106703029332755,
-1.21694480617947));
#34563=CARTESIAN_POINT('Ctrl Pts',(-7.11794122797236,0.412965871424674,
-1.21341531854822));
#34564=CARTESIAN_POINT('Ctrl Pts',(-7.09411770039994,0.81333664327713,-0.99066271615481));
#34565=CARTESIAN_POINT('Ctrl Pts',(-7.07029417282752,1.02843750508761,-0.650686201737506));
#34566=CARTESIAN_POINT('Ctrl Pts',(-7.04647064525511,1.24353836689809,-0.310709687320199));
#34567=CARTESIAN_POINT('Ctrl Pts',(-7.0226471176827,1.27336931866659,0.146490739121003));
#34568=CARTESIAN_POINT('Ctrl Pts',(-6.99882359011028,1.10426763327177,0.511536654314946));
#34569=CARTESIAN_POINT('Ctrl Pts',(-6.97500006253787,0.935165947876942,
0.876582569508885));
#34570=CARTESIAN_POINT('Ctrl Pts',(-6.95117653496545,0.567131625318796,
1.14947397345556));
#34571=CARTESIAN_POINT('Ctrl Pts',(-6.92735300739304,0.168705643738918,
1.20524384305627));
#34572=CARTESIAN_POINT('Ctrl Pts',(-6.90352947982062,-0.229720337840963,
1.26101371265697));
#34573=CARTESIAN_POINT('Ctrl Pts',(-6.87970595224821,-0.658537978442577,
1.09966204791169));
#34574=CARTESIAN_POINT('Ctrl Pts',(-6.85588242467579,-0.92137219093613,
0.795077889353162));
#34575=CARTESIAN_POINT('Ctrl Pts',(-6.83888583316718,-1.10888790332011,
0.577776211116059));
#34576=CARTESIAN_POINT('Ctrl Pts',(-6.82188924165856,-1.21191926571901,
0.287570241923624));
#34577=CARTESIAN_POINT('Ctrl Pts',(-6.80489265014995,-1.21436027551958,
-0.00106957681048473));
#34578=CARTESIAN_POINT('Origin',(-3.875,0.,0.));
#34579=CARTESIAN_POINT('',(-6.29010734985006,-1.21698889981248,-7.32665095025398E-5));
#34580=CARTESIAN_POINT('',(-6.35489265014995,-1.21698887272922,7.32242133118944E-5));
#34581=CARTESIAN_POINT('',(-3.875,-1.215,-1.48794586096403E-16));
#34582=CARTESIAN_POINT('Ctrl Pts',(-6.29010734985006,-1.21698889981248,
-7.32665095025398E-5));
#34583=CARTESIAN_POINT('Ctrl Pts',(-6.31369885384504,-1.21664139445038,
0.398323610426177));
#34584=CARTESIAN_POINT('Ctrl Pts',(-6.33729035784002,-1.00225596389633,
0.7970411536321));
#34585=CARTESIAN_POINT('Ctrl Pts',(-6.360881861835,-0.669584224757944,1.01623442508117));
#34586=CARTESIAN_POINT('Ctrl Pts',(-6.38470538940741,-0.333640643051026,
1.23758347290643));
#34587=CARTESIAN_POINT('Ctrl Pts',(-6.40852891697983,0.12292739193656,1.27585962421094));
#34588=CARTESIAN_POINT('Ctrl Pts',(-6.43235244455225,0.49103611136388,1.11353445102204));
#34589=CARTESIAN_POINT('Ctrl Pts',(-6.45617597212467,0.859144830791203,
0.951209277833139));
#34590=CARTESIAN_POINT('Ctrl Pts',(-6.47999949969708,1.13879423465826,0.588282780150836));
#34591=CARTESIAN_POINT('Ctrl Pts',(-6.5038230272695,1.20191983375759,0.190955897270189));
#34592=CARTESIAN_POINT('Ctrl Pts',(-6.52764655484191,1.26504543285693,-0.206370985610454));
#34593=CARTESIAN_POINT('Ctrl Pts',(-6.55147008241433,1.11164722718855,-0.638098253689441));
#34594=CARTESIAN_POINT('Ctrl Pts',(-6.57529360998674,0.811973402978483,
-0.906517865129097));
#34595=CARTESIAN_POINT('Ctrl Pts',(-6.59911713755915,0.512299578768414,
-1.17493747656875));
#34596=CARTESIAN_POINT('Ctrl Pts',(-6.62294066513157,0.0663501360166598,
-1.28004943136908));
#34597=CARTESIAN_POINT('Ctrl Pts',(-6.64676419270399,-0.321653908877025,
-1.17371810067433));
#34598=CARTESIAN_POINT('Ctrl Pts',(-6.67058772027641,-0.709657953770708,
-1.06738676997957));
#34599=CARTESIAN_POINT('Ctrl Pts',(-6.69441124784882,-1.03971660080632,
-0.749612153789738));
#34600=CARTESIAN_POINT('Ctrl Pts',(-6.71823477542124,-1.16068061187102,
-0.36591799112184));
#34601=CARTESIAN_POINT('Ctrl Pts',(-6.72552563356418,-1.19769995933722,
-0.24849374730308));
#34602=CARTESIAN_POINT('Ctrl Pts',(-6.73281649170712,-1.21513590873778,
-0.124895606612254));
#34603=CARTESIAN_POINT('Ctrl Pts',(-6.74010734985006,-1.21414526361761,
-0.00102520398183079));
#34604=CARTESIAN_POINT('Ctrl Pts',(-6.80489265014995,-1.21436027551958,
-0.00106957681048473));
#34605=CARTESIAN_POINT('Ctrl Pts',(-6.79806571408614,-1.21534074374059,
-0.117006091903337));
#34606=CARTESIAN_POINT('Ctrl Pts',(-6.79123877802234,-1.20009248969292,
-0.232689932458696));
#34607=CARTESIAN_POINT('Ctrl Pts',(-6.78441184195854,-1.1675718035762,-0.343295225079648));
#34608=CARTESIAN_POINT('Ctrl Pts',(-6.76058831438612,-1.05408641933721,
-0.729267528582172));
#34609=CARTESIAN_POINT('Ctrl Pts',(-6.73676478681371,-0.730264866473754,
-1.05339548321545));
#34610=CARTESIAN_POINT('Ctrl Pts',(-6.71294125924129,-0.344400251683041,
-1.16724619030599));
#34611=CARTESIAN_POINT('Ctrl Pts',(-6.68911773166888,0.0414643631076694,
-1.28109689739654));
#34612=CARTESIAN_POINT('Ctrl Pts',(-6.66529420409646,0.489372039825632,
-1.18467035694436));
#34613=CARTESIAN_POINT('Ctrl Pts',(-6.64147067652405,0.79420506113041,-0.922124568184181));
#34614=CARTESIAN_POINT('Ctrl Pts',(-6.61764714895163,1.09903808243519,-0.659578779423996));
#34615=CARTESIAN_POINT('Ctrl Pts',(-6.59382362137922,1.26079644832678,-0.230913742355804));
#34616=CARTESIAN_POINT('Ctrl Pts',(-6.5700000938068,1.20540343124301,0.167564747811473));
#34617=CARTESIAN_POINT('Ctrl Pts',(-6.54617656623438,1.15001041415923,0.566043237978747));
#34618=CARTESIAN_POINT('Ctrl Pts',(-6.52235303866197,0.877466014100086,
0.934335181245106));
#34619=CARTESIAN_POINT('Ctrl Pts',(-6.49852951108955,0.512581026296972,
1.10378259911935));
#34620=CARTESIAN_POINT('Ctrl Pts',(-6.47470598351713,0.147696038493855,
1.27323001699359));
#34621=CARTESIAN_POINT('Ctrl Pts',(-6.45088245594472,-0.309529537053229,
1.24383290947571));
#34622=CARTESIAN_POINT('Ctrl Pts',(-6.4270589283723,-0.649710822647686,
1.02905355139116));
#34623=CARTESIAN_POINT('Ctrl Pts',(-6.40323540079989,-0.989892108242138,
0.814274193306606));
#34624=CARTESIAN_POINT('Ctrl Pts',(-6.37941187322747,-1.21302910388396,
0.414112584655379));
#34625=CARTESIAN_POINT('Ctrl Pts',(-6.35558834565506,-1.21693698036283,
0.0118213808785433));
#34626=CARTESIAN_POINT('Ctrl Pts',(-6.35535644715336,-1.21697501967911,
0.00790547349998427));
#34627=CARTESIAN_POINT('Ctrl Pts',(-6.35512454865165,-1.21699228681968,
0.00398936434018253));
#34628=CARTESIAN_POINT('Ctrl Pts',(-6.35489265014995,-1.21698887272922,
7.32242133118944E-5));
#34629=CARTESIAN_POINT('Origin',(-3.875,0.,0.));
#34630=CARTESIAN_POINT('',(-5.84010734985006,-1.21436037857631,0.00106961527518802));
#34631=CARTESIAN_POINT('',(-5.90489265014995,-1.2141452873099,0.00102522403285088));
#34632=CARTESIAN_POINT('',(-3.875,-1.215,-1.48794586096403E-16));
#34633=CARTESIAN_POINT('Ctrl Pts',(-5.84010734985006,-1.21436037857631,
0.00106961527518802));
#34634=CARTESIAN_POINT('Ctrl Pts',(-5.84693416083814,-1.21534082109932,
0.117003935709098));
#34635=CARTESIAN_POINT('Ctrl Pts',(-5.85376097182621,-1.2000931166481,0.232685591943789));
#34636=CARTESIAN_POINT('Ctrl Pts',(-5.86058778281428,-1.16757359504631,
0.343289003077695));
#34637=CARTESIAN_POINT('Ctrl Pts',(-5.88441131038669,-1.05409019542155,
0.729261812249731));
#34638=CARTESIAN_POINT('Ctrl Pts',(-5.9082348379591,-0.730270408341806,
1.05339169431114));
#34639=CARTESIAN_POINT('Ctrl Pts',(-5.93205836553151,-0.344406397450761,
1.16724447863947));
#34640=CARTESIAN_POINT('Ctrl Pts',(-5.95588189310393,0.0414576134402811,
1.28109726296781));
#34641=CARTESIAN_POINT('Ctrl Pts',(-5.97970542067635,0.489365848142625,
1.18467294956306));
#34642=CARTESIAN_POINT('Ctrl Pts',(-6.00352894824877,0.794200262982349,
0.922128722957946));
#34643=CARTESIAN_POINT('Ctrl Pts',(-6.02735247582118,1.09903467782208,0.659584496352827));
#34644=CARTESIAN_POINT('Ctrl Pts',(-6.0511760033936,1.26079527279918,0.230920356547328));
#34645=CARTESIAN_POINT('Ctrl Pts',(-6.07499953096601,1.20540433683121,-0.167558420373342));
#34646=CARTESIAN_POINT('Ctrl Pts',(-6.09882305853843,1.15001340086323,-0.56603719729401));
#34647=CARTESIAN_POINT('Ctrl Pts',(-6.12264658611084,0.877470933950182,
-0.934330611329849));
#34648=CARTESIAN_POINT('Ctrl Pts',(-6.14647011368326,0.512586826446446,
-1.10377995318354));
#34649=CARTESIAN_POINT('Ctrl Pts',(-6.17029364125568,0.147702718942707,
-1.27322929503724));
#34650=CARTESIAN_POINT('Ctrl Pts',(-6.19411716882809,-0.30952302915172,
-1.24383456470878));
#34651=CARTESIAN_POINT('Ctrl Pts',(-6.21794069640051,-0.64970545087747,
-1.02905697905386));
#34652=CARTESIAN_POINT('Ctrl Pts',(-6.24176422397292,-0.98988787260322,
-0.814279393398937));
#34653=CARTESIAN_POINT('Ctrl Pts',(-6.26558775154534,-1.21302696796029,
-0.414118952417547));
#34654=CARTESIAN_POINT('Ctrl Pts',(-6.28941127911776,-1.2169369514257,-0.0118277597538365));
#34655=CARTESIAN_POINT('Ctrl Pts',(-6.28964330269519,-1.21697503177919,
-0.00790974041732449));
#34656=CARTESIAN_POINT('Ctrl Pts',(-6.28987532627263,-1.21699231754445,
-0.00399151897214472));
#34657=CARTESIAN_POINT('Ctrl Pts',(-6.29010734985006,-1.21698889981248,
-7.32665095025398E-5));
#34658=CARTESIAN_POINT('Ctrl Pts',(-6.35489265014995,-1.21698887272922,
7.32242133118944E-5));
#34659=CARTESIAN_POINT('Ctrl Pts',(-6.33130102107924,-1.21664154855489,
-0.3983257502674));
#34660=CARTESIAN_POINT('Ctrl Pts',(-6.30770939200853,-1.00225352412178,
-0.79704521887662));
#34661=CARTESIAN_POINT('Ctrl Pts',(-6.28411776293781,-0.669578881611528,
-1.01623790290697));
#34662=CARTESIAN_POINT('Ctrl Pts',(-6.2602942353654,-0.333634149065464,
-1.2375851840132));
#34663=CARTESIAN_POINT('Ctrl Pts',(-6.23647070779298,0.122934073342565,
-1.2758589473232));
#34664=CARTESIAN_POINT('Ctrl Pts',(-6.21264718022056,0.491041931694761,
-1.11353184948667));
#34665=CARTESIAN_POINT('Ctrl Pts',(-6.18882365264814,0.859149790046959,
-0.951204751650141));
#34666=CARTESIAN_POINT('Ctrl Pts',(-6.16500012507573,1.13879728434332,-0.588276792667072));
#34667=CARTESIAN_POINT('Ctrl Pts',(-6.14117659750332,1.20192080050794,-0.190949592008526));
#34668=CARTESIAN_POINT('Ctrl Pts',(-6.1173530699309,1.26504431667255,0.206377608650018));
#34669=CARTESIAN_POINT('Ctrl Pts',(-6.09352954235848,1.11164385470542,0.638104050984041));
#34670=CARTESIAN_POINT('Ctrl Pts',(-6.06970601478607,0.811968631768357,
0.906522088974185));
#34671=CARTESIAN_POINT('Ctrl Pts',(-6.04588248721365,0.512293408831295,
1.17494012696433));
#34672=CARTESIAN_POINT('Ctrl Pts',(-6.02205895964123,0.066343424924305,
1.2800497606106));
#34673=CARTESIAN_POINT('Ctrl Pts',(-5.99823543206882,-0.321660050735999,
1.17371639214635));
#34674=CARTESIAN_POINT('Ctrl Pts',(-5.9744119044964,-0.709663526396303,
1.06738302368211));
#34675=CARTESIAN_POINT('Ctrl Pts',(-5.95058837692399,-1.03972049380992,
0.749606653107353));
#34676=CARTESIAN_POINT('Ctrl Pts',(-5.92676484935158,-1.16068249382993,
0.365911882482422));
#34677=CARTESIAN_POINT('Ctrl Pts',(-5.91947411628437,-1.19770059078224,
0.24848946704008));
#34678=CARTESIAN_POINT('Ctrl Pts',(-5.91218338321716,-1.21513593053589,
0.124893473920583));
#34679=CARTESIAN_POINT('Ctrl Pts',(-5.90489265014995,-1.2141452873099,0.00102522403285088));
#34680=CARTESIAN_POINT('Origin',(-3.875,0.,0.));
#34681=CARTESIAN_POINT('',(-5.39010734985006,-1.21322636163708,-0.000530816515116744));
#34682=CARTESIAN_POINT('',(-5.45489265014995,-1.21334113603808,-0.000641635778683531));
#34683=CARTESIAN_POINT('',(-3.875,-1.215,-1.48794586096403E-16));
#34684=CARTESIAN_POINT('Ctrl Pts',(-5.39010734985006,-1.21322636163708,
-0.000530816515116744));
#34685=CARTESIAN_POINT('Ctrl Pts',(-5.40399299540364,-1.21229583382079,
0.235833215312909));
#34686=CARTESIAN_POINT('Ctrl Pts',(-5.41787864095721,-1.14570162521325,
0.472681662538362));
#34687=CARTESIAN_POINT('Ctrl Pts',(-5.43176428651079,-1.01687485630836,
0.668611221932072));
#34688=CARTESIAN_POINT('Ctrl Pts',(-5.4555878140832,-0.79584746012218,1.00476651571784));
#34689=CARTESIAN_POINT('Ctrl Pts',(-5.47941134165562,-0.391631796683574,
1.22047264070872));
#34690=CARTESIAN_POINT('Ctrl Pts',(-5.50323486922803,0.0106629538454742,
1.21694771494172));
#34691=CARTESIAN_POINT('Ctrl Pts',(-5.52705839680045,0.412957704374528,
1.21342278917472));
#34692=CARTESIAN_POINT('Ctrl Pts',(-5.55088192437287,0.813331541994021,
0.990666812649834));
#34693=CARTESIAN_POINT('Ctrl Pts',(-5.57470545194528,1.02843463753263,0.65069012272196));
#34694=CARTESIAN_POINT('Ctrl Pts',(-5.5985289795177,1.24353773307125,0.310713432794086));
#34695=CARTESIAN_POINT('Ctrl Pts',(-5.6223525070901,1.27337008652897,-0.146483970536773));
#34696=CARTESIAN_POINT('Ctrl Pts',(-5.64617603466252,1.10427007370218,-0.51153010059119));
#34697=CARTESIAN_POINT('Ctrl Pts',(-5.66999956223494,0.935170060875382,
-0.876576230645603));
#34698=CARTESIAN_POINT('Ctrl Pts',(-5.69382308980737,0.567137681764061,
-1.14947108742358));
#34699=CARTESIAN_POINT('Ctrl Pts',(-5.71764661737978,0.168712105264506,
-1.20524340488892));
#34700=CARTESIAN_POINT('Ctrl Pts',(-5.7414701449522,-0.229713471235052,
-1.26101572235425));
#34701=CARTESIAN_POINT('Ctrl Pts',(-5.7652936725246,-0.658532245122845,
-1.09966550050696));
#34702=CARTESIAN_POINT('Ctrl Pts',(-5.78911720009702,-0.921368125981851,
-0.795082521441981));
#34703=CARTESIAN_POINT('Ctrl Pts',(-5.80611391668136,-1.10888640855265,
-0.57778008561055));
#34704=CARTESIAN_POINT('Ctrl Pts',(-5.82311063326571,-1.21191937007028,
-0.287572151760318));
#34705=CARTESIAN_POINT('Ctrl Pts',(-5.84010734985006,-1.21436037857631,
0.00106961527518802));
#34706=CARTESIAN_POINT('Ctrl Pts',(-5.90489265014995,-1.2141452873099,0.00102522403285088));
#34707=CARTESIAN_POINT('Ctrl Pts',(-5.88835985564474,-1.21189886013553,
-0.27986399550588));
#34708=CARTESIAN_POINT('Ctrl Pts',(-5.87182706113953,-1.11490208679248,
-0.562153217588061));
#34709=CARTESIAN_POINT('Ctrl Pts',(-5.85529426663433,-0.936643782657277,
-0.777028816434906));
#34710=CARTESIAN_POINT('Ctrl Pts',(-5.83147073906191,-0.6797760388382,-1.08666157405219));
#34711=CARTESIAN_POINT('Ctrl Pts',(-5.8076472114895,-0.254173518573637,
-1.25631391861166));
#34712=CARTESIAN_POINT('Ctrl Pts',(-5.78382368391708,0.145260560092642,
-1.20829413924618));
#34713=CARTESIAN_POINT('Ctrl Pts',(-5.76000015634467,0.544694638758927,
-1.16027435988069));
#34714=CARTESIAN_POINT('Ctrl Pts',(-5.73617662877225,0.91796027582693,-0.894582456590248));
#34715=CARTESIAN_POINT('Ctrl Pts',(-5.71235310119983,1.0941217498074,-0.532891127546195));
#34716=CARTESIAN_POINT('Ctrl Pts',(-5.68852957362741,1.27028322378787,-0.171199798502151));
#34717=CARTESIAN_POINT('Ctrl Pts',(-5.664706046055,1.24934053468083,0.286490956295504));
#34718=CARTESIAN_POINT('Ctrl Pts',(-5.64088251848259,1.04088431532232,0.630583221573055));
#34719=CARTESIAN_POINT('Ctrl Pts',(-5.61705899091017,0.832428095963802,
0.974675486850615));
#34720=CARTESIAN_POINT('Ctrl Pts',(-5.59323546333775,0.436458346353827,
1.20516926260807));
#34721=CARTESIAN_POINT('Ctrl Pts',(-5.56941193576534,0.0343080586227004,
1.21651071279303));
#34722=CARTESIAN_POINT('Ctrl Pts',(-5.54558840819292,-0.36784222910842,
1.22785216297799));
#34723=CARTESIAN_POINT('Ctrl Pts',(-5.52176488062051,-0.776173054960685,
1.02004128759047));
#34724=CARTESIAN_POINT('Ctrl Pts',(-5.49794135304809,-1.00369071422132,
0.68824436605509));
#34725=CARTESIAN_POINT('Ctrl Pts',(-5.48359178541538,-1.14073087459529,
0.488393930328221));
#34726=CARTESIAN_POINT('Ctrl Pts',(-5.46924221778267,-1.21217228758971,
0.243561541831228));
#34727=CARTESIAN_POINT('Ctrl Pts',(-5.45489265014995,-1.21334113603808,
-0.000641635778683531));
#34728=CARTESIAN_POINT('Origin',(-3.875,0.,0.));
#34729=CARTESIAN_POINT('',(-4.94010734985006,-1.21630354408558,-0.000802320355120511));
#34730=CARTESIAN_POINT('',(-5.00489265014995,-1.21648875695904,-0.000697868307776));
#34731=CARTESIAN_POINT('',(-3.875,-1.215,-1.48794586096403E-16));
#34732=CARTESIAN_POINT('Ctrl Pts',(-4.94010734985006,-1.21630354408558,
-0.000802320355120511));
#34733=CARTESIAN_POINT('Ctrl Pts',(-4.96105182996914,-1.21360198855398,
0.353421363843449));
#34734=CARTESIAN_POINT('Ctrl Pts',(-4.98199631008822,-1.0499189859206,0.709819131320941));
#34735=CARTESIAN_POINT('Ctrl Pts',(-5.00294079020731,-0.777920094248849,
0.935903716441848));
#34736=CARTESIAN_POINT('Ctrl Pts',(-5.02676431777972,-0.468531985374048,
1.19306609606182));
#34737=CARTESIAN_POINT('Ctrl Pts',(-5.05058784535213,-0.0190029011941928,
1.28162702087502));
#34738=CARTESIAN_POINT('Ctrl Pts',(-5.07441137292455,0.36480685212754,1.16103031834945));
#34739=CARTESIAN_POINT('Ctrl Pts',(-5.09823490049697,0.748616605449275,
1.04043361582388));
#34740=CARTESIAN_POINT('Ctrl Pts',(-5.12205842806939,1.06670702791289,0.710679285959532));
#34741=CARTESIAN_POINT('Ctrl Pts',(-5.1458819556418,1.17340969880785,0.322777195956391));
#34742=CARTESIAN_POINT('Ctrl Pts',(-5.16970548321422,1.28011236970281,-0.0651248940467475));
#34743=CARTESIAN_POINT('Ctrl Pts',(-5.19352901078663,1.17542728902912,-0.511174744188683));
#34744=CARTESIAN_POINT('Ctrl Pts',(-5.21735253835905,0.907294631330801,
-0.811105351630773));
#34745=CARTESIAN_POINT('Ctrl Pts',(-5.24117606593146,0.639161973632482,
-1.11103595907287));
#34746=CARTESIAN_POINT('Ctrl Pts',(-5.26499959350388,0.207581738909531,
-1.26484732381511));
#34747=CARTESIAN_POINT('Ctrl Pts',(-5.28882312107629,-0.18980538087671,
-1.20210205759585));
#34748=CARTESIAN_POINT('Ctrl Pts',(-5.31264664864871,-0.587192500662953,
-1.13935679137658));
#34749=CARTESIAN_POINT('Ctrl Pts',(-5.33647017622113,-0.950386505512486,
-0.860054894195808));
#34750=CARTESIAN_POINT('Ctrl Pts',(-5.36029370379354,-1.11306394347038,
-0.492101714315088));
#34751=CARTESIAN_POINT('Ctrl Pts',(-5.37023158581238,-1.18092413674523,
-0.338611628558619));
#34752=CARTESIAN_POINT('Ctrl Pts',(-5.38016946783122,-1.21389233540243,
-0.169695285876029));
#34753=CARTESIAN_POINT('Ctrl Pts',(-5.39010734985006,-1.21322636163708,
-0.000530816515116744));
#34754=CARTESIAN_POINT('Ctrl Pts',(-5.45489265014995,-1.21334113603808,
-0.000641635778683531));
#34755=CARTESIAN_POINT('Ctrl Pts',(-5.44541869021025,-1.21411284036108,
-0.161870962058142));
#34756=CARTESIAN_POINT('Ctrl Pts',(-5.43594473027055,-1.1842528333953,-0.322826016203698));
#34757=CARTESIAN_POINT('Ctrl Pts',(-5.42647077033085,-1.12241602959814,
-0.470380286280767));
#34758=CARTESIAN_POINT('Ctrl Pts',(-5.40264724275843,-0.966919193045314,
-0.841425049398009));
#34759=CARTESIAN_POINT('Ctrl Pts',(-5.37882371518601,-0.609221027270653,
-1.12773160794927));
#34760=CARTESIAN_POINT('Ctrl Pts',(-5.3550001876136,-0.21312818352657,-1.19818685296113));
#34761=CARTESIAN_POINT('Ctrl Pts',(-5.33117666004118,0.182964660217511,
-1.268642097973));
#34762=CARTESIAN_POINT('Ctrl Pts',(-5.30735313246877,0.617452181931014,
-1.12324602944548));
#34763=CARTESIAN_POINT('Ctrl Pts',(-5.28352960489635,0.891362307521405,
-0.828582279530157));
#34764=CARTESIAN_POINT('Ctrl Pts',(-5.25970607732393,1.1652724331118,-0.533918529614831));
#34765=CARTESIAN_POINT('Ctrl Pts',(-5.23588254975151,1.27860516257908,-0.0899870983117007));
#34766=CARTESIAN_POINT('Ctrl Pts',(-5.2120590221791,1.17946016019986,0.299915134200719));
#34767=CARTESIAN_POINT('Ctrl Pts',(-5.18823549460669,1.08031515782065,0.689817366713137));
#34768=CARTESIAN_POINT('Ctrl Pts',(-5.16441196703427,0.76869242359494,1.02569040043484));
#34769=CARTESIAN_POINT('Ctrl Pts',(-5.14058843946186,0.387298522532,1.15372232866756));
#34770=CARTESIAN_POINT('Ctrl Pts',(-5.11676491188944,0.00590462146906182,
1.28175425690027));
#34771=CARTESIAN_POINT('Ctrl Pts',(-5.09294138431702,-0.445260446431109,
1.20194507964399));
#34772=CARTESIAN_POINT('Ctrl Pts',(-5.0691178567446,-0.759587181857625,
0.950843136578795));
#34773=CARTESIAN_POINT('Ctrl Pts',(-5.04770945454638,-1.0420488430541,0.725196813902441));
#34774=CARTESIAN_POINT('Ctrl Pts',(-5.02630105234817,-1.21401002870781,
0.361227173945358));
#34775=CARTESIAN_POINT('Ctrl Pts',(-5.00489265014995,-1.21648875695904,
-0.000697868307776));
#34776=CARTESIAN_POINT('Origin',(-3.875,0.,0.));
#34777=CARTESIAN_POINT('',(-4.49010734985006,-1.21569869268569,0.00101898845098317));
#34778=CARTESIAN_POINT('',(-4.55489265014995,-1.21546413760631,0.00106646674887225));
#34779=CARTESIAN_POINT('',(-3.875,-1.215,-1.48794586096403E-16));
#34780=CARTESIAN_POINT('Ctrl Pts',(-4.49010734985006,-1.21569869268569,
0.00101898845098317));
#34781=CARTESIAN_POINT('Ctrl Pts',(-4.49428713696223,-1.21633390645148,
0.0718012148764551));
#34782=CARTESIAN_POINT('Ctrl Pts',(-4.4984669240744,-1.21068428894374,0.142482134878694));
#34783=CARTESIAN_POINT('Ctrl Pts',(-4.50264671118658,-1.19838922396478,
0.211987517016677));
#34784=CARTESIAN_POINT('Ctrl Pts',(-4.52647023875899,-1.12831105690268,
0.608147259931254));
#34785=CARTESIAN_POINT('Ctrl Pts',(-4.55029376633141,-0.842345119511607,
0.966117813998743));
#34786=CARTESIAN_POINT('Ctrl Pts',(-4.57411729390382,-0.471448534467992,
1.12196778867924));
#34787=CARTESIAN_POINT('Ctrl Pts',(-4.59794082147624,-0.100551949424372,
1.27781776335974));
#34788=CARTESIAN_POINT('Ctrl Pts',(-4.62176434904865,0.355275283271792,
1.23154715865325));
#34789=CARTESIAN_POINT('Ctrl Pts',(-4.64558787662107,0.68728864189162,1.00434543968327));
#34790=CARTESIAN_POINT('Ctrl Pts',(-4.66941140419349,1.01930200051144,0.777143720713295));
#34791=CARTESIAN_POINT('Ctrl Pts',(-4.6932349317659,1.22750148505493,0.369010887479842));
#34792=CARTESIAN_POINT('Ctrl Pts',(-4.71705845933832,1.21654285387123,-0.0331500253492225));
#34793=CARTESIAN_POINT('Ctrl Pts',(-4.74088198691073,1.20558422268752,-0.435310938178298));
#34794=CARTESIAN_POINT('Ctrl Pts',(-4.76470551448314,0.9754674757766,-0.831499930602986));
#34795=CARTESIAN_POINT('Ctrl Pts',(-4.78852904205556,0.63157379010677,-1.04028360899131));
#34796=CARTESIAN_POINT('Ctrl Pts',(-4.81235256962798,0.287680104436951,
-1.24906728737962));
#34797=CARTESIAN_POINT('Ctrl Pts',(-4.83617609720039,-0.169990519991771,
-1.27044565173157));
#34798=CARTESIAN_POINT('Ctrl Pts',(-4.85999962477281,-0.531849386513239,
-1.09462855323224));
#34799=CARTESIAN_POINT('Ctrl Pts',(-4.88382315234523,-0.893708253034712,
-0.918811454732897));
#34800=CARTESIAN_POINT('Ctrl Pts',(-4.90764667991764,-1.15975536164893,
-0.545798893382257));
#34801=CARTESIAN_POINT('Ctrl Pts',(-4.93147020749006,-1.20815534917116,
-0.146410695493564));
#34802=CARTESIAN_POINT('Ctrl Pts',(-4.93434925494339,-1.21400443513854,
-0.0981450652031645));
#34803=CARTESIAN_POINT('Ctrl Pts',(-4.93722830239672,-1.21667490238758,
-0.0494942329786094));
#34804=CARTESIAN_POINT('Ctrl Pts',(-4.94010734985006,-1.21630354408558,
-0.000802320355120511));
#34805=CARTESIAN_POINT('Ctrl Pts',(-5.00489265014995,-1.21648875695904,
-0.000697868307776));
#34806=CARTESIAN_POINT('Ctrl Pts',(-5.00247752477575,-1.2167683873322,-0.0415273680999158));
#34807=CARTESIAN_POINT('Ctrl Pts',(-5.00006239940156,-1.21489108992725,
-0.0823308472073769));
#34808=CARTESIAN_POINT('Ctrl Pts',(-4.99764727402736,-1.21077218381049,
-0.122906778219102));
#34809=CARTESIAN_POINT('Ctrl Pts',(-4.97382374645495,-1.17014204738398,
-0.523160041077697));
#34810=CARTESIAN_POINT('Ctrl Pts',(-4.95000021888253,-0.911393371578093,
-0.901271857920772));
#34811=CARTESIAN_POINT('Ctrl Pts',(-4.92617669131011,-0.553019227242496,
-1.08408721582794));
#34812=CARTESIAN_POINT('Ctrl Pts',(-4.9023531637377,-0.194645082906902,
-1.26690257373511));
#34813=CARTESIAN_POINT('Ctrl Pts',(-4.87852963616528,0.263354529958394,
-1.25442147270637));
#34814=CARTESIAN_POINT('Ctrl Pts',(-4.85470610859287,0.611240255558246,
-1.05235959025731));
#34815=CARTESIAN_POINT('Ctrl Pts',(-4.83088258102045,0.959125981158095,
-0.850297707808241));
#34816=CARTESIAN_POINT('Ctrl Pts',(-4.80705905344803,1.1968978194925,-0.458655043938839));
#34817=CARTESIAN_POINT('Ctrl Pts',(-4.78323552587562,1.21566897066551,-0.0567830166731548));
#34818=CARTESIAN_POINT('Ctrl Pts',(-4.7594119983032,1.23444012183852,0.345089010592532));
#34819=CARTESIAN_POINT('Ctrl Pts',(-4.73558847073079,1.03421058585014,0.757190401254506));
#34820=CARTESIAN_POINT('Ctrl Pts',(-4.71176494315838,0.706674793677344,
0.990800733347795));
#34821=CARTESIAN_POINT('Ctrl Pts',(-4.68794141558596,0.379139001504556,
1.22441106544108));
#34822=CARTESIAN_POINT('Ctrl Pts',(-4.66411788801354,-0.0757030468526306,
1.27953033896569));
#34823=CARTESIAN_POINT('Ctrl Pts',(-4.64029436044113,-0.449557991462852,
1.13091687118609));
#34824=CARTESIAN_POINT('Ctrl Pts',(-4.61647083286871,-0.823412936073079,
0.982303403406478));
#34825=CARTESIAN_POINT('Ctrl Pts',(-4.59264730529629,-1.11628077693633,
0.62995719432264));
#34826=CARTESIAN_POINT('Ctrl Pts',(-4.56882377772388,-1.19404368829401,
0.235233984931332));
#34827=CARTESIAN_POINT('Ctrl Pts',(-4.56418006853257,-1.20920132374984,
0.158294086341503));
#34828=CARTESIAN_POINT('Ctrl Pts',(-4.55953635934126,-1.21618620842765,
0.0797441053466365));
#34829=CARTESIAN_POINT('Ctrl Pts',(-4.55489265014995,-1.21546413760631,
0.00106646674887225));
#34830=CARTESIAN_POINT('Origin',(-3.875,0.,0.));
#34831=CARTESIAN_POINT('',(-4.04010734985006,-1.21302894219882,0.000187577549479595));
#34832=CARTESIAN_POINT('',(-4.10489265014995,-1.21300507934972,5.85455518045706E-5));
#34833=CARTESIAN_POINT('',(-3.875,-1.215,-1.48794586096403E-16));
#34834=CARTESIAN_POINT('Ctrl Pts',(-4.04010734985006,-1.21302894219882,
0.000187577549479595));
#34835=CARTESIAN_POINT('Ctrl Pts',(-4.05134597152774,-1.21329263069357,
0.191571241354318));
#34836=CARTESIAN_POINT('Ctrl Pts',(-4.06258459320541,-1.17069438186556,
0.382843920803326));
#34837=CARTESIAN_POINT('Ctrl Pts',(-4.07382321488309,-1.08461318382743,
0.551987029696823));
#34838=CARTESIAN_POINT('Ctrl Pts',(-4.09764674245551,-0.902139046540549,
0.910535046880482));
#34839=CARTESIAN_POINT('Ctrl Pts',(-4.12147027002792,-0.524273698081696,
1.16964354415799));
#34840=CARTESIAN_POINT('Ctrl Pts',(-4.14529379760034,-0.124059282017878,
1.21065467166778));
#34841=CARTESIAN_POINT('Ctrl Pts',(-4.16911732517275,0.276155134045952,
1.25166579917756));
#34842=CARTESIAN_POINT('Ctrl Pts',(-4.19294085274517,0.698718617714743,
1.07457955691961));
#34843=CARTESIAN_POINT('Ctrl Pts',(-4.21676438031759,0.950119667324172,
0.760491983685306));
#34844=CARTESIAN_POINT('Ctrl Pts',(-4.24058790789,1.20152071693359,0.446404410451012));
#34845=CARTESIAN_POINT('Ctrl Pts',(-4.26441143546242,1.28175933248366,-0.00468449375963097));
#34846=CARTESIAN_POINT('Ctrl Pts',(-4.28823496303483,1.154090514497,-0.386200108536821));
#34847=CARTESIAN_POINT('Ctrl Pts',(-4.31205849060725,1.02642169651034,-0.767715723314017));
#34848=CARTESIAN_POINT('Ctrl Pts',(-4.33588201817967,0.690845444986967,
-1.07965804865777));
#34849=CARTESIAN_POINT('Ctrl Pts',(-4.35970554575208,0.301037756232491,
-1.1791741638996));
#34850=CARTESIAN_POINT('Ctrl Pts',(-4.3835290733245,-0.0887699325219851,
-1.27869027914143));
#34851=CARTESIAN_POINT('Ctrl Pts',(-4.40735260089691,-0.532809058507552,
-1.16578018428134));
#34852=CARTESIAN_POINT('Ctrl Pts',(-4.43117612846932,-0.827733423133778,
-0.892150670970461));
#34853=CARTESIAN_POINT('Ctrl Pts',(-4.45081986892957,-1.07091393687214,
-0.666528872292524));
#34854=CARTESIAN_POINT('Ctrl Pts',(-4.47046360938981,-1.21271337931513,
-0.331636155886707));
#34855=CARTESIAN_POINT('Ctrl Pts',(-4.49010734985006,-1.21569869268569,
0.00101898845098317));
#34856=CARTESIAN_POINT('Ctrl Pts',(-4.55489265014995,-1.21546413760631,
0.00106646674887225));
#34857=CARTESIAN_POINT('Ctrl Pts',(-4.53571283176884,-1.21248178306146,
-0.323894196546626));
#34858=CARTESIAN_POINT('Ctrl Pts',(-4.51653301338774,-1.07802484522109,
-0.651032597879852));
#34859=CARTESIAN_POINT('Ctrl Pts',(-4.49735319500663,-0.844912941184178,
-0.87589809854854));
#34860=CARTESIAN_POINT('Ctrl Pts',(-4.47352966743422,-0.555361300864557,
-1.15520676293833));
#34861=CARTESIAN_POINT('Ctrl Pts',(-4.4497061398618,-0.113600038373203,
-1.27672388201915));
#34862=CARTESIAN_POINT('Ctrl Pts',(-4.42588261228938,0.278067787493538,
-1.18480110684447));
#34863=CARTESIAN_POINT('Ctrl Pts',(-4.40205908471697,0.669735613360282,
-1.0928783316698));
#34864=CARTESIAN_POINT('Ctrl Pts',(-4.37823555714455,1.01131000260242,-0.787515662239641));
#34865=CARTESIAN_POINT('Ctrl Pts',(-4.35441202957214,1.14636813226695,-0.408552888307276));
#34866=CARTESIAN_POINT('Ctrl Pts',(-4.33058850199972,1.28142626193149,-0.0295901143749137));
#34867=CARTESIAN_POINT('Ctrl Pts',(-4.3067649744273,1.20996813201843,0.422972764059648));
#34868=CARTESIAN_POINT('Ctrl Pts',(-4.28294144685489,0.964717748647626,
0.741886125133569));
#34869=CARTESIAN_POINT('Ctrl Pts',(-4.25911791928247,0.719467365276819,
1.06079948620749));
#34870=CARTESIAN_POINT('Ctrl Pts',(-4.23529439171006,0.300424728448258,
1.24606332992077));
#34871=CARTESIAN_POINT('Ctrl Pts',(-4.21147086413764,-0.100511019938621,
1.2128367128729));
#34872=CARTESIAN_POINT('Ctrl Pts',(-4.18764733656523,-0.501446768325502,
1.17961009582503));
#34873=CARTESIAN_POINT('Ctrl Pts',(-4.16382380899281,-0.884275628270695,
0.927893018016035));
#34874=CARTESIAN_POINT('Ctrl Pts',(-4.14000028142039,-1.0736824331033,0.572958454049525));
#34875=CARTESIAN_POINT('Ctrl Pts',(-4.12829773766358,-1.16672245056733,
0.398608234377028));
#34876=CARTESIAN_POINT('Ctrl Pts',(-4.11659519390676,-1.21309068378989,
0.199352146337624));
#34877=CARTESIAN_POINT('Ctrl Pts',(-4.10489265014995,-1.21300507934972,
5.85455518045706E-5));
#34878=CARTESIAN_POINT('Origin',(-3.875,0.,0.));
#34879=CARTESIAN_POINT('',(-3.59010734985006,-1.21500971925273,-0.00111129482518957));
#34880=CARTESIAN_POINT('',(-3.65489265014995,-1.21524902215508,-0.00109519578050164));
#34881=CARTESIAN_POINT('',(-3.875,-1.215,-1.48794586096403E-16));
#34882=CARTESIAN_POINT('Ctrl Pts',(-3.59010734985006,-1.21500971925273,
-0.00111129482518957));
#34883=CARTESIAN_POINT('Ctrl Pts',(-3.60840480609324,-1.21215498276526,
0.309197329221224));
#34884=CARTESIAN_POINT('Ctrl Pts',(-3.62670226233643,-1.09101085463479,
0.62148703039356));
#34885=CARTESIAN_POINT('Ctrl Pts',(-3.64499971857961,-0.87670201402857,
0.844078798504059));
#34886=CARTESIAN_POINT('Ctrl Pts',(-3.66882324615202,-0.597669097904114,
1.13389619467622));
#34887=CARTESIAN_POINT('Ctrl Pts',(-3.69264677372444,-0.160699812471054,
1.27165423805471));
#34888=CARTESIAN_POINT('Ctrl Pts',(-3.71647030129685,0.234097252973719,
1.19426710397464));
#34889=CARTESIAN_POINT('Ctrl Pts',(-3.74029382886927,0.628894318418485,
1.11687996989456));
#34890=CARTESIAN_POINT('Ctrl Pts',(-3.76411735644169,0.981519163874969,
0.824347658355936));
#34891=CARTESIAN_POINT('Ctrl Pts',(-3.7879408840141,1.13048844777284,0.45063434061106));
#34892=CARTESIAN_POINT('Ctrl Pts',(-3.81176441158652,1.27945773167071,0.0769210228661713));
#34893=CARTESIAN_POINT('Ctrl Pts',(-3.83558793915893,1.22477145400996,-0.377973301084966));
#34894=CARTESIAN_POINT('Ctrl Pts',(-3.85941146673135,0.99147300855165,-0.705731331881578));
#34895=CARTESIAN_POINT('Ctrl Pts',(-3.88323499430376,0.758174563093346,
-1.03348936267818));
#34896=CARTESIAN_POINT('Ctrl Pts',(-3.90705852187618,0.34626394983749,-1.23411110032026));
#34897=CARTESIAN_POINT('Ctrl Pts',(-3.93088204944859,-0.0556257751113993,
-1.21572250642532));
#34898=CARTESIAN_POINT('Ctrl Pts',(-3.95470557702101,-0.457515500060289,
-1.19733391253038));
#34899=CARTESIAN_POINT('Ctrl Pts',(-3.97852910459343,-0.849384336702215,
-0.959934987098434));
#34900=CARTESIAN_POINT('Ctrl Pts',(-4.00235263216584,-1.05177729196572,
-0.612241755837557));
#34901=CARTESIAN_POINT('Ctrl Pts',(-4.01493753806058,-1.15869245337526,
-0.428570946283624));
#34902=CARTESIAN_POINT('Ctrl Pts',(-4.02752244395532,-1.21273366623107,
-0.214122100972612));
#34903=CARTESIAN_POINT('Ctrl Pts',(-4.04010734985006,-1.21302894219882,
0.000187577549479595));
#34904=CARTESIAN_POINT('Ctrl Pts',(-4.10489265014995,-1.21300507934972,
5.85455518045706E-5));
#34905=CARTESIAN_POINT('Ctrl Pts',(-4.09277166633435,-1.21291641400863,
-0.206361063712259));
#34906=CARTESIAN_POINT('Ctrl Pts',(-4.08065068251875,-1.16299248122336,
-0.412820916319921));
#34907=CARTESIAN_POINT('Ctrl Pts',(-4.06852969870315,-1.06347545239199,
-0.59168853240628));
#34908=CARTESIAN_POINT('Ctrl Pts',(-4.04470617113073,-0.867876917128068,
-0.943248904771545));
#34909=CARTESIAN_POINT('Ctrl Pts',(-4.02088264355831,-0.480695096880224,
-1.18821759937806));
#34910=CARTESIAN_POINT('Ctrl Pts',(-3.9970591159859,-0.0792385815975481,
-1.21441204062207));
#34911=CARTESIAN_POINT('Ctrl Pts',(-3.97323558841348,0.322217933685125,
-1.24060648186608));
#34912=CARTESIAN_POINT('Ctrl Pts',(-3.94941206084107,0.737949144002628,
-1.04802666974759));
#34913=CARTESIAN_POINT('Ctrl Pts',(-3.92558853326865,0.97757236389716,-0.724863870368748));
#34914=CARTESIAN_POINT('Ctrl Pts',(-3.90176500569624,1.21719558379169,-0.401701070989909));
#34915=CARTESIAN_POINT('Ctrl Pts',(-3.87794147812382,1.28071081326325,0.0520447156492849));
#34916=CARTESIAN_POINT('Ctrl Pts',(-3.85411795055141,1.13903147027479,0.428582158920665));
#34917=CARTESIAN_POINT('Ctrl Pts',(-3.83029442297899,0.997352127286321,
0.805119602192056));
#34918=CARTESIAN_POINT('Ctrl Pts',(-3.80647089540658,0.650478211837817,
1.10444870209563));
#34919=CARTESIAN_POINT('Ctrl Pts',(-3.78264736783416,0.257259446777643,
1.18949272140064));
#34920=CARTESIAN_POINT('Ctrl Pts',(-3.75882384026174,-0.135959318282526,
1.27453674070565));
#34921=CARTESIAN_POINT('Ctrl Pts',(-3.73500031268933,-0.575522932954362,
1.14529567941211));
#34922=CARTESIAN_POINT('Ctrl Pts',(-3.71117678511691,-0.860134743741845,
0.860955039377548));
#34923=CARTESIAN_POINT('Ctrl Pts',(-3.69241540679459,-1.0842707303607,0.637032603714567));
#34924=CARTESIAN_POINT('Ctrl Pts',(-3.67365402847227,-1.21230879822748,
0.316920602375664));
#34925=CARTESIAN_POINT('Ctrl Pts',(-3.65489265014995,-1.21524902215508,
-0.00109519578050164));
#34926=CARTESIAN_POINT('Origin',(-3.875,0.,0.));
#34927=CARTESIAN_POINT('',(-3.14010734985006,-1.21677568176215,0.000466761158960617));
#34928=CARTESIAN_POINT('',(-3.20489265014995,-1.21663669410215,0.000593093442031073));
#34929=CARTESIAN_POINT('',(-3.875,-1.215,-1.48794586096403E-16));
#34930=CARTESIAN_POINT('Ctrl Pts',(-3.14010734985006,-1.21677568176215,
0.000466761158960617));
#34931=CARTESIAN_POINT('Ctrl Pts',(-3.14164011308633,-1.21690273304476,
0.0263631226345996));
#34932=CARTESIAN_POINT('Ctrl Pts',(-3.1431728763226,-1.21614766855925,0.0522519381467224));
#34933=CARTESIAN_POINT('Ctrl Pts',(-3.14470563955888,-1.21448695277727,
0.0780825269799757));
#34934=CARTESIAN_POINT('Ctrl Pts',(-3.16852916713129,-1.18867467643506,
0.479563806487453));
#34935=CARTESIAN_POINT('Ctrl Pts',(-3.19235269470371,-0.94407465143364,
0.866978652223446));
#34936=CARTESIAN_POINT('Ctrl Pts',(-3.21617622227613,-0.592700622392402,
1.0629117610138));
#34937=CARTESIAN_POINT('Ctrl Pts',(-3.23999974984854,-0.241326593351153,
1.25884486980417));
#34938=CARTESIAN_POINT('Ctrl Pts',(-3.26382327742096,0.216821439729918,
1.26329624164888));
#34939=CARTESIAN_POINT('Ctrl Pts',(-3.28764680499337,0.571936152525624,
1.07422738604077));
#34940=CARTESIAN_POINT('Ctrl Pts',(-3.31147033256579,0.927050865321321,
0.885158530432671));
#34941=CARTESIAN_POINT('Ctrl Pts',(-3.3352938601382,1.17913225783166,0.502569447371758));
#34942=CARTESIAN_POINT('Ctrl Pts',(-3.35911738771062,1.21274051878192,0.101665498525122));
#34943=CARTESIAN_POINT('Ctrl Pts',(-3.38294091528303,1.24634877973219,-0.299238450321518));
#34944=CARTESIAN_POINT('Ctrl Pts',(-3.40676444285545,1.06148390912237,-0.718457264953887));
#34945=CARTESIAN_POINT('Ctrl Pts',(-3.43058797042787,0.74280414198523,-0.964011123450032));
#34946=CARTESIAN_POINT('Ctrl Pts',(-3.45441149800028,0.424124374848083,
-1.20956498194618));
#34947=CARTESIAN_POINT('Ctrl Pts',(-3.4782350255727,-0.0283702888163973,
-1.28145388430611));
#34948=CARTESIAN_POINT('Ctrl Pts',(-3.50205855314511,-0.407461465865948,
-1.14675655364169));
#34949=CARTESIAN_POINT('Ctrl Pts',(-3.52588208071753,-0.786552642915494,
-1.01205922297728));
#34950=CARTESIAN_POINT('Ctrl Pts',(-3.54970560828994,-1.09224033335011,
-0.670775659288539));
#34951=CARTESIAN_POINT('Ctrl Pts',(-3.57352913586236,-1.18453590515949,
-0.279195502961247));
#34952=CARTESIAN_POINT('Ctrl Pts',(-3.57905520719159,-1.20594465378586,
-0.188365130825994));
#34953=CARTESIAN_POINT('Ctrl Pts',(-3.58458127852083,-1.21587188704514,
-0.0948285617373963));
#34954=CARTESIAN_POINT('Ctrl Pts',(-3.59010734985006,-1.21500971925273,
-0.00111129482518957));
#34955=CARTESIAN_POINT('Ctrl Pts',(-3.65489265014995,-1.21524902215508,
-0.00109519578050164));
#34956=CARTESIAN_POINT('Ctrl Pts',(-3.64983050089985,-1.21604234618994,
-0.0869014412757421));
#34957=CARTESIAN_POINT('Ctrl Pts',(-3.64476835164976,-1.20772835783292,
-0.172555080006382));
#34958=CARTESIAN_POINT('Ctrl Pts',(-3.63970620239967,-1.1897374078851,-0.25612547218169));
#34959=CARTESIAN_POINT('Ctrl Pts',(-3.61588267482725,-1.10506825433774,
-0.649425124930798));
#34960=CARTESIAN_POINT('Ctrl Pts',(-3.59205914725483,-0.806069940339887,
-0.996584211653431));
#34961=CARTESIAN_POINT('Ctrl Pts',(-3.56823561968242,-0.429667720848445,
-1.13862241629187));
#34962=CARTESIAN_POINT('Ctrl Pts',(-3.54441209211,-0.0532655013570036,-1.28066062093032));
#34963=CARTESIAN_POINT('Ctrl Pts',(-3.52058856453759,0.400540623628025,
-1.21757794348457));
#34964=CARTESIAN_POINT('Ctrl Pts',(-3.49676503696517,0.723931691739427,
-0.978262880271319));
#34965=CARTESIAN_POINT('Ctrl Pts',(-3.47294150939276,1.04732275985083,-0.73894781705807));
#34966=CARTESIAN_POINT('Ctrl Pts',(-3.44911798182034,1.2402987710886,-0.323400368077314));
#34967=CARTESIAN_POINT('Ctrl Pts',(-3.42529445424792,1.21448702131941,0.0780809340886104));
#34968=CARTESIAN_POINT('Ctrl Pts',(-3.40147092667551,1.18867527155022,0.479562236254538));
#34969=CARTESIAN_POINT('Ctrl Pts',(-3.37764739910309,0.944075760774064,
0.866977391605637));
#34970=CARTESIAN_POINT('Ctrl Pts',(-3.35382387153068,0.592701998122636,
1.06291095518057));
#34971=CARTESIAN_POINT('Ctrl Pts',(-3.33000034395826,0.241328235471213,
1.25884451875551));
#34972=CARTESIAN_POINT('Ctrl Pts',(-3.30617681638584,-0.216819779055476,
1.26329649055428));
#34973=CARTESIAN_POINT('Ctrl Pts',(-3.28235328881343,-0.57193472962917,
1.07422810532282));
#34974=CARTESIAN_POINT('Ctrl Pts',(-3.25852976124101,-0.927049680202874,
0.885159720091348));
#34975=CARTESIAN_POINT('Ctrl Pts',(-3.2347062336686,-1.17913156682357,0.502570977829626));
#34976=CARTESIAN_POINT('Ctrl Pts',(-3.21088270609618,-1.21274035194041,
0.101667084136921));
#34977=CARTESIAN_POINT('Ctrl Pts',(-3.20888602078077,-1.21555715425936,
0.0680667319223174));
#34978=CARTESIAN_POINT('Ctrl Pts',(-3.20688933546536,-1.2168393216259,0.0343377273868962));
#34979=CARTESIAN_POINT('Ctrl Pts',(-3.20489265014995,-1.21663669410215,
0.000593093442031074));
#34980=CARTESIAN_POINT('Origin',(-3.875,0.,0.));
#34981=CARTESIAN_POINT('',(-2.69010734985006,-1.21361800699981,0.000827517035146899));
#34982=CARTESIAN_POINT('',(-2.75489265014995,-1.21346326955177,0.000734265906742561));
#34983=CARTESIAN_POINT('',(-3.875,-1.215,-1.48794586096403E-16));
#34984=CARTESIAN_POINT('Ctrl Pts',(-2.69010734985006,-1.21361800699981,
0.000827517035146899));
#34985=CARTESIAN_POINT('Ctrl Pts',(-2.69869894765184,-1.21453325658579,
0.146957062172633));
#34986=CARTESIAN_POINT('Ctrl Pts',(-2.70729054545362,-1.19012564930912,
0.292791146029));
#34987=CARTESIAN_POINT('Ctrl Pts',(-2.71588214325539,-1.13903094055414,
0.428583662714895));
#34988=CARTESIAN_POINT('Ctrl Pts',(-2.73970567082781,-0.997351100446097,
0.805120930872916));
#34989=CARTESIAN_POINT('Ctrl Pts',(-2.76352919840022,-0.650476783306341,
1.10444958475712));
#34990=CARTESIAN_POINT('Ctrl Pts',(-2.78735272597264,-0.257257895936303,
1.18949309138987));
#34991=CARTESIAN_POINT('Ctrl Pts',(-2.81117625354506,0.135960991433729,
1.27453659802261));
#34992=CARTESIAN_POINT('Ctrl Pts',(-2.83499978111747,0.575524449034037,
1.1452949574039));
#34993=CARTESIAN_POINT('Ctrl Pts',(-2.85882330868989,0.860135895298941,
0.860953936691222));
#34994=CARTESIAN_POINT('Ctrl Pts',(-2.8826468362623,1.14474734156385,0.576612915978538));
#34995=CARTESIAN_POINT('Ctrl Pts',(-2.90647036383472,1.27440677649335,0.137172515171866));
#34996=CARTESIAN_POINT('Ctrl Pts',(-2.93029389140714,1.18973710545467,-0.256127037600748));
#34997=CARTESIAN_POINT('Ctrl Pts',(-2.95411741897955,1.105067434416,-0.649426590373356));
#34998=CARTESIAN_POINT('Ctrl Pts',(-2.97794094655197,0.806068657409177,
-0.996585295111915));
#34999=CARTESIAN_POINT('Ctrl Pts',(-3.00176447412438,0.429666241424461,
-1.13862301068702));
#35000=CARTESIAN_POINT('Ctrl Pts',(-3.0255880016968,0.0532638254397441,
-1.28066072626213));
#35001=CARTESIAN_POINT('Ctrl Pts',(-3.04941152926921,-0.400542229522857,
-1.21757745267379));
#35002=CARTESIAN_POINT('Ctrl Pts',(-3.07323505684163,-0.723932993162663,
-0.97826195924014));
#35003=CARTESIAN_POINT('Ctrl Pts',(-3.09552582117777,-1.0265173723596,-0.754343597448325));
#35004=CARTESIAN_POINT('Ctrl Pts',(-3.11781658551391,-1.21492799248291,
-0.376140451981686));
#35005=CARTESIAN_POINT('Ctrl Pts',(-3.14010734985006,-1.21677568176215,
0.000466761158960617));
#35006=CARTESIAN_POINT('Ctrl Pts',(-3.20489265014995,-1.21663669410215,
0.000593093442031074));
#35007=CARTESIAN_POINT('Ctrl Pts',(-3.18306580789294,-1.21442166353939,
-0.368287669315083));
#35008=CARTESIAN_POINT('Ctrl Pts',(-3.16123896563594,-1.03477582261886,
-0.739036123563579));
#35009=CARTESIAN_POINT('Ctrl Pts',(-3.13941212337893,-0.742805384007626,
-0.96401012375946));
#35010=CARTESIAN_POINT('Ctrl Pts',(-3.11558859580652,-0.424125947345048,
-1.20956439283947));
#35011=CARTESIAN_POINT('Ctrl Pts',(-3.0917650682341,0.0283686095930635,
-1.2814538858758));
#35012=CARTESIAN_POINT('Ctrl Pts',(-3.06794154066169,0.40745995253944,-1.14675705548211));
#35013=CARTESIAN_POINT('Ctrl Pts',(-3.04411801308927,0.786551295485811,
-1.01206022508842));
#35014=CARTESIAN_POINT('Ctrl Pts',(-3.02029448551685,1.09223942444044,-0.670777071264702));
#35015=CARTESIAN_POINT('Ctrl Pts',(-2.99647095794444,1.18453550657428,-0.279197046700459));
#35016=CARTESIAN_POINT('Ctrl Pts',(-2.97264743037202,1.27683158870812,0.112382977863789));
#35017=CARTESIAN_POINT('Ctrl Pts',(-2.94882390279961,1.15573562402117,0.55425987316857));
#35018=CARTESIAN_POINT('Ctrl Pts',(-2.92500037522719,0.876703095246122,
0.844077626766233));
#35019=CARTESIAN_POINT('Ctrl Pts',(-2.90117684765478,0.59767056647107,1.1338953803639));
#35020=CARTESIAN_POINT('Ctrl Pts',(-2.87735332008236,0.160701473607927,
1.27165399225445));
#35021=CARTESIAN_POINT('Ctrl Pts',(-2.85352979250994,-0.234095682233161,
1.19426737742485));
#35022=CARTESIAN_POINT('Ctrl Pts',(-2.82970626493753,-0.628892838074238,
1.11688076259526));
#35023=CARTESIAN_POINT('Ctrl Pts',(-2.80588273736512,-0.981518056893257,
0.82434892104552));
#35024=CARTESIAN_POINT('Ctrl Pts',(-2.7820592097927,-1.1304878261398,0.450635808798139));
#35025=CARTESIAN_POINT('Ctrl Pts',(-2.77300368991178,-1.18711246759842,
0.308584363753787));
#35026=CARTESIAN_POINT('Ctrl Pts',(-2.76394817003087,-1.21431250172664,
0.154803662174065));
#35027=CARTESIAN_POINT('Ctrl Pts',(-2.75489265014995,-1.21346326955177,
0.000734265906742561));
#35028=CARTESIAN_POINT('Origin',(-3.875,0.,0.));
#35029=CARTESIAN_POINT('',(-2.24010734985006,-1.21377365198237,-0.000902035925798433));
#35030=CARTESIAN_POINT('',(-2.30489265014994,-1.21396226950007,-0.000972860349384481));
#35031=CARTESIAN_POINT('',(-3.875,-1.215,-1.48794586096403E-16));
#35032=CARTESIAN_POINT('Ctrl Pts',(-2.24010734985006,-1.21377365198237,
-0.000902035925798433));
#35033=CARTESIAN_POINT('Ctrl Pts',(-2.25575778221734,-1.21194130236611,
0.265201375550419));
#35034=CARTESIAN_POINT('Ctrl Pts',(-2.27140821458463,-1.12582985342833,
0.532383292654391));
#35035=CARTESIAN_POINT('Ctrl Pts',(-2.28705864695191,-0.9647168037228,0.741887409314856));
#35036=CARTESIAN_POINT('Ctrl Pts',(-2.31088217452433,-0.719465995830789,
1.06080045801943));
#35037=CARTESIAN_POINT('Ctrl Pts',(-2.33470570209674,-0.300423104710086,
1.24606375801843));
#35038=CARTESIAN_POINT('Ctrl Pts',(-2.35852922966916,0.100512611290855,
1.21283661490585));
#35039=CARTESIAN_POINT('Ctrl Pts',(-2.38235275724157,0.501448327291784,
1.17960947179328));
#35040=CARTESIAN_POINT('Ctrl Pts',(-2.40617628481399,0.884276868172959,
0.927891885569145));
#35041=CARTESIAN_POINT('Ctrl Pts',(-2.4299998123864,1.07368321337605,0.572957063662786));
#35042=CARTESIAN_POINT('Ctrl Pts',(-2.45382333995882,1.26308955857914,0.218022241756422));
#35043=CARTESIAN_POINT('Ctrl Pts',(-2.47764686753124,1.25907370810414,-0.24012981583216));
#35044=CARTESIAN_POINT('Ctrl Pts',(-2.50147039510365,1.06347470693787,-0.591689941767681));
#35045=CARTESIAN_POINT('Ctrl Pts',(-2.52529392267607,0.867875705771602,
-0.943250067703207));
#35046=CARTESIAN_POINT('Ctrl Pts',(-2.54911745024848,0.480693553914047,
-1.18821826198566));
#35047=CARTESIAN_POINT('Ctrl Pts',(-2.5729409778209,0.0792369931733729,
-1.21441217813333));
#35048=CARTESIAN_POINT('Ctrl Pts',(-2.59676450539331,-0.32221956756729,
-1.24060609428099));
#35049=CARTESIAN_POINT('Ctrl Pts',(-2.62058803296573,-0.737950537191079,
-1.04802573229389));
#35050=CARTESIAN_POINT('Ctrl Pts',(-2.64441156053814,-0.977573340464803,
-0.724862610084428));
#35051=CARTESIAN_POINT('Ctrl Pts',(-2.65964349030878,-1.13077977472665,
-0.518243419580755));
#35052=CARTESIAN_POINT('Ctrl Pts',(-2.67487542007942,-1.21199537315011,
-0.258243615052597));
#35053=CARTESIAN_POINT('Ctrl Pts',(-2.69010734985006,-1.21361800699981,
0.000827517035146899));
#35054=CARTESIAN_POINT('Ctrl Pts',(-2.75489265014995,-1.21346326955177,
0.000734265906742561));
#35055=CARTESIAN_POINT('Ctrl Pts',(-2.74012464245845,-1.21207831678756,
-0.250526628997279));
#35056=CARTESIAN_POINT('Ctrl Pts',(-2.72535663476695,-1.13609341191021,
-0.502555337563078));
#35057=CARTESIAN_POINT('Ctrl Pts',(-2.71058862707545,-0.991473905375597,
-0.705730013660128));
#35058=CARTESIAN_POINT('Ctrl Pts',(-2.68676509950303,-0.758175895690786,
-1.03348834092597));
#35059=CARTESIAN_POINT('Ctrl Pts',(-2.66294157193062,-0.346265556647109,
-1.23411061251262));
#35060=CARTESIAN_POINT('Ctrl Pts',(-2.63911804435821,0.0556241812254146,
-1.21572254551951));
#35061=CARTESIAN_POINT('Ctrl Pts',(-2.61529451678579,0.457513919097938,
-1.1973344785264));
#35062=CARTESIAN_POINT('Ctrl Pts',(-2.59147098921337,0.849383055799309,
-0.959936072953527));
#35063=CARTESIAN_POINT('Ctrl Pts',(-2.56764746164095,1.05177646084693,-0.612243116441262));
#35064=CARTESIAN_POINT('Ctrl Pts',(-2.54382393406854,1.25416986589456,-0.264550159929002));
#35065=CARTESIAN_POINT('Ctrl Pts',(-2.52000040649613,1.26708753928845,0.193437347522645));
#35066=CARTESIAN_POINT('Ctrl Pts',(-2.49617687892371,1.08461387669191,0.551985593751234));
#35067=CARTESIAN_POINT('Ctrl Pts',(-2.4723533513513,0.902140214095379,0.910533839979817));
#35068=CARTESIAN_POINT('Ctrl Pts',(-2.44852982377888,0.524275215508423,
1.16964282498534));
#35069=CARTESIAN_POINT('Ctrl Pts',(-2.42470629620646,0.124060864275674,
1.21065447555299));
#35070=CARTESIAN_POINT('Ctrl Pts',(-2.40088276863405,-0.276153486957087,
1.25166612612065));
#35071=CARTESIAN_POINT('Ctrl Pts',(-2.37705924106163,-0.69871719083565,
1.07458044225042));
#35072=CARTESIAN_POINT('Ctrl Pts',(-2.35323571348922,-0.950118644851876,
0.760493207021673));
#35073=CARTESIAN_POINT('Ctrl Pts',(-2.33712135904279,-1.12016785885049,
0.548043013817145));
#35074=CARTESIAN_POINT('Ctrl Pts',(-2.32100700459637,-1.21190627045042,
0.272911350689318));
#35075=CARTESIAN_POINT('Ctrl Pts',(-2.30489265014994,-1.21396226950007,
-0.000972860349384481));
#35076=CARTESIAN_POINT('Origin',(-3.875,0.,0.));
#35077=CARTESIAN_POINT('',(-1.79010734985006,-1.21687501168408,-0.000345202031853675));
#35078=CARTESIAN_POINT('',(-1.85489265014995,-1.21695226826403,-0.000204119252572796));
#35079=CARTESIAN_POINT('',(-3.875,-1.215,-1.48794586096403E-16));
#35080=CARTESIAN_POINT('Ctrl Pts',(-1.79010734985006,-1.21687501168408,
-0.000345202031853675));
#35081=CARTESIAN_POINT('Ctrl Pts',(-1.81281661678285,-1.21543111614067,
0.383249301044499));
#35082=CARTESIAN_POINT('Ctrl Pts',(-1.83552588371564,-1.01889028811385,
0.768118048257717));
#35083=CARTESIAN_POINT('Ctrl Pts',(-1.85823515064843,-0.706673515517428,
0.990801686492171));
#35084=CARTESIAN_POINT('Ctrl Pts',(-1.88205867822084,-0.379137408229808,
1.22441159609891));
#35085=CARTESIAN_POINT('Ctrl Pts',(-1.90588220579326,0.0757047248680525,
1.27953027534214));
#35086=CARTESIAN_POINT('Ctrl Pts',(-1.92970573336567,0.449559485187943,
1.13091631374865));
#35087=CARTESIAN_POINT('Ctrl Pts',(-1.95352926093809,0.823414245507845,
0.982302352155159));
#35088=CARTESIAN_POINT('Ctrl Pts',(-1.97735278851051,1.11628163304977,0.629955749724934));
#35089=CARTESIAN_POINT('Ctrl Pts',(-2.00117631608292,1.19404402957313,0.235232427526729));
#35090=CARTESIAN_POINT('Ctrl Pts',(-2.02499984365534,1.27180642609648,-0.159490894671465));
#35091=CARTESIAN_POINT('Ctrl Pts',(-2.04882337122775,1.13446383160127,-0.596590936637636));
#35092=CARTESIAN_POINT('Ctrl Pts',(-2.07264689880017,0.844911817399206,
-0.87589922953649));
#35093=CARTESIAN_POINT('Ctrl Pts',(-2.09647042637258,0.555359803197147,
-1.15520752243534));
#35094=CARTESIAN_POINT('Ctrl Pts',(-2.120293953945,0.11359836928824,-1.27672406626688));
#35095=CARTESIAN_POINT('Ctrl Pts',(-2.14411748151742,-0.27806934705301,
-1.18480077553459));
#35096=CARTESIAN_POINT('Ctrl Pts',(-2.16794100908983,-0.669737063394275,
-1.09287748480229));
#35097=CARTESIAN_POINT('Ctrl Pts',(-2.19176453666225,-1.01131106216788,
-0.787514359506141));
#35098=CARTESIAN_POINT('Ctrl Pts',(-2.21558806423466,-1.14636869922301,
-0.408551398152983));
#35099=CARTESIAN_POINT('Ctrl Pts',(-2.2237611594398,-1.19270268240313,-0.278541249448389));
#35100=CARTESIAN_POINT('Ctrl Pts',(-2.23193425464493,-1.21473055639954,
-0.139868708881864));
#35101=CARTESIAN_POINT('Ctrl Pts',(-2.24010734985006,-1.21377365198237,
-0.000902035925798433));
#35102=CARTESIAN_POINT('Ctrl Pts',(-2.30489265014994,-1.21396226950007,
-0.000972860349384481));
#35103=CARTESIAN_POINT('Ctrl Pts',(-2.29718347702395,-1.21494586786098,
-0.13200018796546));
#35104=CARTESIAN_POINT('Ctrl Pts',(-2.28947430389796,-1.19540380974007,
-0.262742010627656));
#35105=CARTESIAN_POINT('Ctrl Pts',(-2.28176513077197,-1.15409098828612,
-0.386198586194984));
#35106=CARTESIAN_POINT('Ctrl Pts',(-2.25794160319955,-1.02642267355024,
-0.767714357595668));
#35107=CARTESIAN_POINT('Ctrl Pts',(-2.23411807562714,-0.690846839924569,
-1.07965711380979));
#35108=CARTESIAN_POINT('Ctrl Pts',(-2.21029454805472,-0.301039292341793,
-1.17917373685424));
#35109=CARTESIAN_POINT('Ctrl Pts',(-2.18647102048231,0.0887682552409884,
-1.27869035989869));
#35110=CARTESIAN_POINT('Ctrl Pts',(-2.16264749290989,0.532807516780883,
-1.16578084977346));
#35111=CARTESIAN_POINT('Ctrl Pts',(-2.13882396533747,0.827732231614367,
-0.892151730350494));
#35112=CARTESIAN_POINT('Ctrl Pts',(-2.11500043776506,1.12265694644784,-0.618522610927539));
#35113=CARTESIAN_POINT('Ctrl Pts',(-2.09117691019264,1.26846711457492,-0.184173882206858));
#35114=CARTESIAN_POINT('Ctrl Pts',(-2.06735338262023,1.1983894683434,0.211985941492073));
#35115=CARTESIAN_POINT('Ctrl Pts',(-2.04352985504781,1.12831182211188,0.608145765191016));
#35116=CARTESIAN_POINT('Ctrl Pts',(-2.01970632747539,0.842346361521747,
0.966116683868196));
#35117=CARTESIAN_POINT('Ctrl Pts',(-1.99588279990298,0.471449990912945,
1.12196714001866));
#35118=CARTESIAN_POINT('Ctrl Pts',(-1.97205927233056,0.100553620304143,
1.27781759616912));
#35119=CARTESIAN_POINT('Ctrl Pts',(-1.94823574475815,-0.355273660323328,
1.23154758979285));
#35120=CARTESIAN_POINT('Ctrl Pts',(-1.92441221718573,-0.687287307315033,
1.00434631199737));
#35121=CARTESIAN_POINT('Ctrl Pts',(-1.9012390281738,-1.01023759135217,0.783347211922782));
#35122=CARTESIAN_POINT('Ctrl Pts',(-1.87806583916187,-1.21604174683208,
0.391160195305395));
#35123=CARTESIAN_POINT('Ctrl Pts',(-1.85489265014995,-1.21695226826403,
-0.000204119252572796));
#35124=CARTESIAN_POINT('Origin',(-3.875,0.,0.));
#35125=CARTESIAN_POINT('',(-1.34010734985006,-1.2147956596487,0.00111167046010718));
#35126=CARTESIAN_POINT('',(-1.40489265014995,-1.21456320713733,0.00109666547093623));
#35127=CARTESIAN_POINT('',(-3.875,-1.215,-1.48794586096403E-16));
#35128=CARTESIAN_POINT('Ctrl Pts',(-1.34010734985006,-1.2147956596487,0.00111167046010718));
#35129=CARTESIAN_POINT('Ctrl Pts',(-1.34605192377594,-1.2157089644333,0.101971735915578));
#35130=CARTESIAN_POINT('Ctrl Pts',(-1.35199649770182,-1.20419912218747,
0.202626225854525));
#35131=CARTESIAN_POINT('Ctrl Pts',(-1.3579410716277,-1.17945980404156,0.299916684419064));
#35132=CARTESIAN_POINT('Ctrl Pts',(-1.38176459920011,-1.08031429162624,
0.689818795326428));
#35133=CARTESIAN_POINT('Ctrl Pts',(-1.40558812677253,-0.768691101236954,
1.02569143594608));
#35134=CARTESIAN_POINT('Ctrl Pts',(-1.42941165434494,-0.387297020092423,
1.15372286954436));
#35135=CARTESIAN_POINT('Ctrl Pts',(-1.45323518191736,-0.00590293894791455,
1.28175430314263));
#35136=CARTESIAN_POINT('Ctrl Pts',(-1.47705870948977,0.44526203295183,1.20194452971952));
#35137=CARTESIAN_POINT('Ctrl Pts',(-1.50088223706219,0.759588447271108,
0.950842167264673));
#35138=CARTESIAN_POINT('Ctrl Pts',(-1.52470576463461,1.07391486159039,0.699739804809822));
#35139=CARTESIAN_POINT('Ctrl Pts',(-1.54852929220702,1.25140271832922,0.277344853323226));
#35140=CARTESIAN_POINT('Ctrl Pts',(-1.57235281977944,1.21077205702477,-0.122908367057554));
#35141=CARTESIAN_POINT('Ctrl Pts',(-1.59617634735185,1.17014139572032,-0.523161587438345));
#35142=CARTESIAN_POINT('Ctrl Pts',(-1.61999987492427,0.911392216372567,
-0.90127307671332));
#35143=CARTESIAN_POINT('Ctrl Pts',(-1.64382340249668,0.553017822372426,
-1.0840879705008));
#35144=CARTESIAN_POINT('Ctrl Pts',(-1.6676469300691,0.194643428372295,-1.26690286428827));
#35145=CARTESIAN_POINT('Ctrl Pts',(-1.69147045764152,-0.263356180280222,
-1.25442116258826));
#35146=CARTESIAN_POINT('Ctrl Pts',(-1.71529398521393,-0.611241650744325,
-1.05235881876606));
#35147=CARTESIAN_POINT('Ctrl Pts',(-1.73911751278635,-0.959127121208428,
-0.85029647494387));
#35148=CARTESIAN_POINT('Ctrl Pts',(-1.76294104035876,-1.19689845348412,
-0.458653488999493));
#35149=CARTESIAN_POINT('Ctrl Pts',(-1.78676456793118,-1.21566907888328,
-0.0567814260421754));
#35150=CARTESIAN_POINT('Ctrl Pts',(-1.7878788285708,-1.21654700802286,-0.0379852918190725));
#35151=CARTESIAN_POINT('Ctrl Pts',(-1.78899308921043,-1.21694585835547,
-0.0191667808005626));
#35152=CARTESIAN_POINT('Ctrl Pts',(-1.79010734985006,-1.21687501168408,
-0.000345202031853675));
#35153=CARTESIAN_POINT('Ctrl Pts',(-1.85489265014995,-1.21695226826403,
-0.000204119252572796));
#35154=CARTESIAN_POINT('Ctrl Pts',(-1.85424231158946,-1.21697782138048,
-0.0111874718168012));
#35155=CARTESIAN_POINT('Ctrl Pts',(-1.85359197302897,-1.21684199964081,
-0.0221701764183581));
#35156=CARTESIAN_POINT('Ctrl Pts',(-1.85294163446849,-1.21654286351776,
-0.0331484310200425));
#35157=CARTESIAN_POINT('Ctrl Pts',(-1.82911810689607,-1.20558475937286,
-0.435309347027362));
#35158=CARTESIAN_POINT('Ctrl Pts',(-1.80529457932365,-0.975468537727084,
-0.831498629827334));
#35159=CARTESIAN_POINT('Ctrl Pts',(-1.78147105175124,-0.631575135093402,
-1.04028275285737));
#35160=CARTESIAN_POINT('Ctrl Pts',(-1.75764752417882,-0.287681732459729,
-1.24906687588741));
#35161=CARTESIAN_POINT('Ctrl Pts',(-1.7338239966064,0.169988851161846,-1.27044583914752));
#35162=CARTESIAN_POINT('Ctrl Pts',(-1.71000046903399,0.531847937959752,
-1.09462921946797));
#35163=CARTESIAN_POINT('Ctrl Pts',(-1.68617694146157,0.893707024757658,
-0.918812599788423));
#35164=CARTESIAN_POINT('Ctrl Pts',(-1.66235341388916,1.15975461473189,-0.545800397169212));
#35165=CARTESIAN_POINT('Ctrl Pts',(-1.63852988631674,1.20815512394341,-0.146412273808625));
#35166=CARTESIAN_POINT('Ctrl Pts',(-1.61470635874433,1.25655563315493,0.252975849551963));
#35167=CARTESIAN_POINT('Ctrl Pts',(-1.59088283117191,1.08730906160373,0.678739893653927));
#35168=CARTESIAN_POINT('Ctrl Pts',(-1.5670593035995,0.777921298304252,0.935902671445341));
#35169=CARTESIAN_POINT('Ctrl Pts',(-1.54323577602708,0.46853353500476,1.19306544923676));
#35170=CARTESIAN_POINT('Ctrl Pts',(-1.51941224845466,0.0190045799569751,
1.28162696071762));
#35171=CARTESIAN_POINT('Ctrl Pts',(-1.49558872088225,-0.364805320954119,
1.16103076409948));
#35172=CARTESIAN_POINT('Ctrl Pts',(-1.47176519330983,-0.748615221865207,
1.04043456748134));
#35173=CARTESIAN_POINT('Ctrl Pts',(-1.44794166573742,-1.06670606863961,
0.710680662764208));
#35174=CARTESIAN_POINT('Ctrl Pts',(-1.424118138165,-1.17340924408634,0.322778723580791));
#35175=CARTESIAN_POINT('Ctrl Pts',(-1.41770964215998,-1.20211225087217,
0.218433637823035));
#35176=CARTESIAN_POINT('Ctrl Pts',(-1.41130114615496,-1.21551919148474,
0.109880945361187));
#35177=CARTESIAN_POINT('Ctrl Pts',(-1.40489265014995,-1.21456320713733,
0.00109666547093623));
#35178=CARTESIAN_POINT('Origin',(-3.875,0.,0.));
#35179=CARTESIAN_POINT('',(-0.890107349850054,-1.21307144811218,-0.000301679661677823));
#35180=CARTESIAN_POINT('',(-0.954892650149944,-1.21314228096755,-0.000424764636864103));
#35181=CARTESIAN_POINT('',(-3.875,-1.215,-1.48794586096403E-16));
#35182=CARTESIAN_POINT('Ctrl Pts',(-0.890107349850054,-1.21307144811218,
-0.000301679661677823));
#35183=CARTESIAN_POINT('Ctrl Pts',(-0.903110758341441,-1.21257958185045,
0.221115114836065));
#35184=CARTESIAN_POINT('Ctrl Pts',(-0.916114166832826,-1.15466388054098,
0.442771501567673));
#35185=CARTESIAN_POINT('Ctrl Pts',(-0.929117575324213,-1.04088370137469,
0.630584464127237));
#35186=CARTESIAN_POINT('Ctrl Pts',(-0.952941102896628,-0.832427184965302,
0.974676345495014));
#35187=CARTESIAN_POINT('Ctrl Pts',(-0.976764630469044,-0.436456767496894,
1.20516987715727));
#35188=CARTESIAN_POINT('Ctrl Pts',(-1.00058815804146,-0.034306369757509,
1.21651086436758));
#35189=CARTESIAN_POINT('Ctrl Pts',(-1.02441168561388,0.367844027981887,
1.22785185157789));
#35190=CARTESIAN_POINT('Ctrl Pts',(-1.04823521318629,0.776174405992254,
1.02004029433626));
#35191=CARTESIAN_POINT('Ctrl Pts',(-1.07205874075871,1.00369159274397,0.688243032164823));
#35192=CARTESIAN_POINT('Ctrl Pts',(-1.09588226833112,1.23120877949568,0.356445769993402));
#35193=CARTESIAN_POINT('Ctrl Pts',(-1.11970579590354,1.27791277498875,-0.09933719710782));
#35194=CARTESIAN_POINT('Ctrl Pts',(-1.14352932347595,1.12241547143391,-0.470381749254917));
#35195=CARTESIAN_POINT('Ctrl Pts',(-1.16735285104837,0.966918167879057,
-0.84142630140202));
#35196=CARTESIAN_POINT('Ctrl Pts',(-1.19117637862078,0.60921956527629,-1.12773243859501));
#35197=CARTESIAN_POINT('Ctrl Pts',(-1.2149999061932,0.213126605972733,-1.1981871760399));
#35198=CARTESIAN_POINT('Ctrl Pts',(-1.23882343376562,-0.182966353330836,
-1.26864191348479));
#35199=CARTESIAN_POINT('Ctrl Pts',(-1.26264696133803,-0.61745366933519,
-1.12324525118158));
#35200=CARTESIAN_POINT('Ctrl Pts',(-1.28647048891045,-0.891363410116701,
-0.828581129432447));
#35201=CARTESIAN_POINT('Ctrl Pts',(-1.30434944255699,-1.09692572845437,
-0.607443174189));
#35202=CARTESIAN_POINT('Ctrl Pts',(-1.32222839620352,-1.21204879601934,
-0.302235963457676));
#35203=CARTESIAN_POINT('Ctrl Pts',(-1.34010734985006,-1.2147956596487,0.00111167046010718));
#35204=CARTESIAN_POINT('Ctrl Pts',(-1.40489265014995,-1.21456320713733,
0.00109666547093623));
#35205=CARTESIAN_POINT('Ctrl Pts',(-1.38747761858255,-1.21196532807569,
-0.294523658992334));
#35206=CARTESIAN_POINT('Ctrl Pts',(-1.37006258701515,-1.10330071711548,
-0.591854200681401));
#35207=CARTESIAN_POINT('Ctrl Pts',(-1.35264755544775,-0.907295667300257,
-0.811104140109695));
#35208=CARTESIAN_POINT('Ctrl Pts',(-1.32882402787534,-0.639163410948359,
-1.11103509096706));
#35209=CARTESIAN_POINT('Ctrl Pts',(-1.30500050030292,-0.207583394125489,
-1.2648470190321));
#35210=CARTESIAN_POINT('Ctrl Pts',(-1.28117697273051,0.189803798807097,
-1.20210227400952));
#35211=CARTESIAN_POINT('Ctrl Pts',(-1.25735344515809,0.587190991739688,
-1.13935752898695));
#35212=CARTESIAN_POINT('Ctrl Pts',(-1.23352991758568,0.950385360781995,
-0.860056110876766));
#35213=CARTESIAN_POINT('Ctrl Pts',(-1.20970639001326,1.11306327236761,-0.492103156261569));
#35214=CARTESIAN_POINT('Ctrl Pts',(-1.18588286244084,1.27574118395322,-0.124150201646372));
#35215=CARTESIAN_POINT('Ctrl Pts',(-1.16205933486843,1.23790263808214,0.332454289473836));
#35216=CARTESIAN_POINT('Ctrl Pts',(-1.13823580729601,1.01687569553182,0.668609867168432));
#35217=CARTESIAN_POINT('Ctrl Pts',(-1.1144122797236,0.795848752981512,1.00476544486302));
#35218=CARTESIAN_POINT('Ctrl Pts',(-1.09058875215118,0.391633413751968,
1.22047210913201));
#35219=CARTESIAN_POINT('Ctrl Pts',(-1.06676522457877,-0.0106613438959427,
1.21694770327565));
#35220=CARTESIAN_POINT('Ctrl Pts',(-1.04294169700635,-0.412956101543859,
1.21342329741929));
#35221=CARTESIAN_POINT('Ctrl Pts',(-1.01911816943393,-0.813330277610143,
0.990667821437577));
#35222=CARTESIAN_POINT('Ctrl Pts',(-0.995294641861518,-1.02843378651698,
0.650691436184902));
#35223=CARTESIAN_POINT('Ctrl Pts',(-0.981827311290994,-1.15003081082509,
0.458504349178061));
#35224=CARTESIAN_POINT('Ctrl Pts',(-0.968359980720469,-1.21242294632906,
0.228858278483662));
#35225=CARTESIAN_POINT('Ctrl Pts',(-0.954892650149944,-1.21314228096755,
-0.000424764636864103));
#35226=CARTESIAN_POINT('Origin',(-3.875,0.,0.));
#35227=CARTESIAN_POINT('',(-0.440107349850056,-1.21588398405722,-0.000947377684412109));
#35228=CARTESIAN_POINT('',(-0.504892650149942,-1.2161173910499,-0.000883162254970131));
#35229=CARTESIAN_POINT('',(-3.875,-1.215,-1.48794586096403E-16));
#35230=CARTESIAN_POINT('Ctrl Pts',(-0.440107349850056,-1.21588398405722,
-0.000947377684412109));
#35231=CARTESIAN_POINT('Ctrl Pts',(-0.460169592906947,-1.21293866576822,
0.338647307153245));
#35232=CARTESIAN_POINT('Ctrl Pts',(-0.480231835963839,-1.06433222539992,
0.680481871379908));
#35233=CARTESIAN_POINT('Ctrl Pts',(-0.50029407902073,-0.811976032752873,
0.906516706944358));
#35234=CARTESIAN_POINT('Ctrl Pts',(-0.524117606593145,-0.512307910073469,
1.17492872458993));
#35235=CARTESIAN_POINT('Ctrl Pts',(-0.547941134165561,-0.0663411673267536,
1.2800503233636));
#35236=CARTESIAN_POINT('Ctrl Pts',(-0.571764661737977,0.321666109547873,
1.17371941224906));
#35237=CARTESIAN_POINT('Ctrl Pts',(-0.595588189310392,0.709673386422499,
1.06738850113453));
#35238=CARTESIAN_POINT('Ctrl Pts',(-0.619411716882807,1.03972119742504,
0.749605080131778));
#35239=CARTESIAN_POINT('Ctrl Pts',(-0.643235244455223,1.16068062812135,
0.365908576638235));
#35240=CARTESIAN_POINT('Ctrl Pts',(-0.667058772027639,1.28164005881766,
-0.0177879268553193));
#35241=CARTESIAN_POINT('Ctrl Pts',(-0.690882299600056,1.19351110920773,
-0.467397512839677));
#35242=CARTESIAN_POINT('Ctrl Pts',(-0.714705827172472,0.936644043228513,
-0.777029118824175));
#35243=CARTESIAN_POINT('Ctrl Pts',(-0.738529354744887,0.679776977249306,
-1.08666072480866));
#35244=CARTESIAN_POINT('Ctrl Pts',(-0.762352882317302,0.254171794900829,
-1.2563143507933));
#35245=CARTESIAN_POINT('Ctrl Pts',(-0.786176409889718,-0.145262806446263,
-1.20829448088716));
#35246=CARTESIAN_POINT('Ctrl Pts',(-0.809999937462134,-0.54469740779336,
-1.16027461098102));
#35247=CARTESIAN_POINT('Ctrl Pts',(-0.83382346503455,-0.917961428139059,
-0.894581245184098));
#35248=CARTESIAN_POINT('Ctrl Pts',(-0.857646992606965,-1.09412213063674,
-0.532889446748983));
#35249=CARTESIAN_POINT('Ctrl Pts',(-0.868467111687995,-1.17413042380949,
-0.368617035041528));
#35250=CARTESIAN_POINT('Ctrl Pts',(-0.879287230769025,-1.21348072938081,
-0.184542302771571));
#35251=CARTESIAN_POINT('Ctrl Pts',(-0.890107349850054,-1.21307144811218,
-0.000301679661677823));
#35252=CARTESIAN_POINT('Ctrl Pts',(-0.954892650149944,-1.21314228096755,
-0.000424764636864103));
#35253=CARTESIAN_POINT('Ctrl Pts',(-0.944536453148053,-1.2136954396791,
-0.176740356751778));
#35254=CARTESIAN_POINT('Ctrl Pts',(-0.934180256146162,-1.17777897841535,
-0.352841275988632));
#35255=CARTESIAN_POINT('Ctrl Pts',(-0.92382405914427,-1.10427065644089,
-0.511528610604347));
#35256=CARTESIAN_POINT('Ctrl Pts',(-0.900000531571855,-0.935171175710573,
-0.876574977617282));
#35257=CARTESIAN_POINT('Ctrl Pts',(-0.87617700399944,-0.567139372502564,
-1.14947041711951));
#35258=CARTESIAN_POINT('Ctrl Pts',(-0.852353476427024,-0.168713786606679,
-1.20524320627726));
#35259=CARTESIAN_POINT('Ctrl Pts',(-0.828529948854608,0.2297117992892,-1.26101599543501));
#35260=CARTESIAN_POINT('Ctrl Pts',(-0.804706421282191,0.658531167872964,
-1.09966613424829));
#35261=CARTESIAN_POINT('Ctrl Pts',(-0.780882893709776,0.921367262878983,
-0.795083600172721));
#35262=CARTESIAN_POINT('Ctrl Pts',(-0.75705936613736,1.18420335788501,-0.49050106609715));
#35263=CARTESIAN_POINT('Ctrl Pts',(-0.733235838564946,1.28105617931329,
-0.0426858591327475));
#35264=CARTESIAN_POINT('Ctrl Pts',(-0.70941231099253,1.1675736252803,0.343287263096404));
#35265=CARTESIAN_POINT('Ctrl Pts',(-0.685588783420115,1.0540910712473,0.729260385325549));
#35266=CARTESIAN_POINT('Ctrl Pts',(-0.661765255847698,0.730273141753013,
1.05339142281944));
#35267=CARTESIAN_POINT('Ctrl Pts',(-0.637941728275282,0.344408651243341,
1.16724437696144));
#35268=CARTESIAN_POINT('Ctrl Pts',(-0.614118200702865,-0.0414558392663365,
1.28109733110344));
#35269=CARTESIAN_POINT('Ctrl Pts',(-0.59029467313045,-0.489366890791401,
1.18467220189356));
#35270=CARTESIAN_POINT('Ctrl Pts',(-0.566471145558034,-0.794200427296363,
0.922129012820161));
#35271=CARTESIAN_POINT('Ctrl Pts',(-0.545944980422003,-1.0568426195696,
0.695923853324785));
#35272=CARTESIAN_POINT('Ctrl Pts',(-0.525418815285973,-1.2132724933316,
0.346402432135793));
#35273=CARTESIAN_POINT('Ctrl Pts',(-0.504892650149942,-1.2161173910499,
-0.000883162254970131));
#35274=CARTESIAN_POINT('Origin',(-3.875,0.,0.));
#35275=CARTESIAN_POINT('',(1.11022302462516E-15,-1.215,-1.48794586096403E-16));
#35276=CARTESIAN_POINT('',(-0.0548926501499415,-1.2158567361346,0.000987498914498598));
#35277=CARTESIAN_POINT('',(-3.875,-1.215,-1.48794586096403E-16));
#35278=CARTESIAN_POINT('',(0.,-1.20342780657953,0.167291704370512));
#35279=CARTESIAN_POINT('Origin',(0.,0.,0.));
#35280=CARTESIAN_POINT('Ctrl Pts',(1.10154940724527E-15,-1.20342780657953,
0.167291704370495));
#35281=CARTESIAN_POINT('Ctrl Pts',(-0.0238235275724144,-1.14778002846286,
0.567598962951908));
#35282=CARTESIAN_POINT('Ctrl Pts',(-0.0476470551448301,-0.877196554917926,
0.934492539965354));
#35283=CARTESIAN_POINT('Ctrl Pts',(-0.0714705827172457,-0.512872496153858,
1.10355045672817));
#35284=CARTESIAN_POINT('Ctrl Pts',(-0.095294110289662,-0.148548437389779,
1.27260837349098));
#35285=CARTESIAN_POINT('Ctrl Pts',(-0.119117637862078,0.309516206593437,
1.24383063000316));
#35286=CARTESIAN_POINT('Ctrl Pts',(-0.142941165434494,0.649908400043695,
1.02920423803292));
#35287=CARTESIAN_POINT('Ctrl Pts',(-0.16676469300691,0.990300593493944,
0.814577846062692));
#35288=CARTESIAN_POINT('Ctrl Pts',(-0.190588220579325,1.21302033641124,
0.414102805610063));
#35289=CARTESIAN_POINT('Ctrl Pts',(-0.214411748151741,1.21682758227759,
0.0117367051186408));
#35290=CARTESIAN_POINT('Ctrl Pts',(-0.238235275724156,1.22063482814394,
-0.390629395372782));
#35291=CARTESIAN_POINT('Ctrl Pts',(-0.262058803296572,1.00552957695933,
-0.794886555902997));
#35292=CARTESIAN_POINT('Ctrl Pts',(-0.285882330868987,0.669635953571026,
-1.01619465631964));
#35293=CARTESIAN_POINT('Ctrl Pts',(-0.309705858441404,0.333742330182708,
-1.23750275673629));
#35294=CARTESIAN_POINT('Ctrl Pts',(-0.333529386013819,-0.122939665409323,
-1.27586179703936));
#35295=CARTESIAN_POINT('Ctrl Pts',(-0.357352913586235,-0.491074246481195,
-1.11355454158985));
#35296=CARTESIAN_POINT('Ctrl Pts',(-0.381176441158651,-0.859208827553056,
-0.951247286140343));
#35297=CARTESIAN_POINT('Ctrl Pts',(-0.404999968731066,-1.13879599410476,
-0.588273734938262));
#35298=CARTESIAN_POINT('Ctrl Pts',(-0.428823496303482,-1.20190482607457,
-0.190935741078487));
#35299=CARTESIAN_POINT('Ctrl Pts',(-0.432584780819007,-1.21186851729366,
-0.128203585263544));
#35300=CARTESIAN_POINT('Ctrl Pts',(-0.436346065334531,-1.21643617455966,
-0.0646148462726548));
#35301=CARTESIAN_POINT('Ctrl Pts',(-0.440107349850056,-1.21588398405722,
-0.000947377684412109));
#35302=CARTESIAN_POINT('Ctrl Pts',(-0.504892650149942,-1.2161173910499,
-0.000883162254970131));
#35303=CARTESIAN_POINT('Ctrl Pts',(-0.501595287713558,-1.21657440086199,
-0.0566717845354851));
#35304=CARTESIAN_POINT('Ctrl Pts',(-0.498297925277174,-1.21306802377492,
-0.112402709462593));
#35305=CARTESIAN_POINT('Ctrl Pts',(-0.495000562840789,-1.20540187658012,
-0.167555461232997));
#35306=CARTESIAN_POINT('Ctrl Pts',(-0.471177035268374,-1.15001376787406,
-0.566035497275865));
#35307=CARTESIAN_POINT('Ctrl Pts',(-0.447353507695957,-0.877481528977088,
-0.934334320424685));
#35308=CARTESIAN_POINT('Ctrl Pts',(-0.423529980123542,-0.512593280682101,
-1.10378186225489));
#35309=CARTESIAN_POINT('Ctrl Pts',(-0.399706452551125,-0.147705032387104,
-1.2732294040851));
#35310=CARTESIAN_POINT('Ctrl Pts',(-0.375882924978708,0.309539225305917,
-1.24382566459669));
#35311=CARTESIAN_POINT('Ctrl Pts',(-0.352059397406292,0.649713618299758,
-1.0290528454463));
#35312=CARTESIAN_POINT('Ctrl Pts',(-0.328235869833877,0.989888011293583,
-0.814280026295927));
#35313=CARTESIAN_POINT('Ctrl Pts',(-0.304412342261461,1.21299253958824,
-0.414138127483595));
#35314=CARTESIAN_POINT('Ctrl Pts',(-0.280588814689046,1.21691880955427,
-0.0118387594639543));
#35315=CARTESIAN_POINT('Ctrl Pts',(-0.25676528711663,1.22084507952029,0.390460608555698));
#35316=CARTESIAN_POINT('Ctrl Pts',(-0.232941759544215,1.00559309115768,
0.794917445782652));
#35317=CARTESIAN_POINT('Ctrl Pts',(-0.209118231971799,0.6696198577145,1.01625136658536));
#35318=CARTESIAN_POINT('Ctrl Pts',(-0.185294704399383,0.333646624271334,
1.23758528738806));
#35319=CARTESIAN_POINT('Ctrl Pts',(-0.161471176826967,-0.123047854252383,
1.27579629176651));
#35320=CARTESIAN_POINT('Ctrl Pts',(-0.137647649254552,-0.491099606844063,
1.11350124652694));
#35321=CARTESIAN_POINT('Ctrl Pts',(-0.113824121682136,-0.859151359435747,
0.95120620128737));
#35322=CARTESIAN_POINT('Ctrl Pts',(-0.0900005941097201,-1.1385603860954,
0.588405106429774));
#35323=CARTESIAN_POINT('Ctrl Pts',(-0.0661770665373044,-1.20179772134079,
0.191021162694664));
#35324=CARTESIAN_POINT('Ctrl Pts',(-0.0624155944081834,-1.21178219879999,
0.128278622809408));
#35325=CARTESIAN_POINT('Ctrl Pts',(-0.0586541222790624,-1.21637774826694,
0.0646739696606226));
#35326=CARTESIAN_POINT('Ctrl Pts',(-0.0548926501499415,-1.2158567361346,
0.000987498914498598));
#35327=CARTESIAN_POINT('Origin',(-8.61687266823562,0.,0.));
#35328=CARTESIAN_POINT('',(-0.291872668235618,-0.958947183310973,-0.000747180795175678));
#35329=CARTESIAN_POINT('',(-0.203127331764369,-0.958925693334137,0.000778823732210353));
#35330=CARTESIAN_POINT('',(-8.61687266823562,-0.95825,-1.32069628103871E-13));
#35331=CARTESIAN_POINT('',(-1.1100891904241E-15,0.570663296631698,0.771750790290221));
#35332=CARTESIAN_POINT('Ctrl Pts',(-0.291872668235618,-0.958947183310973,
-0.000747180795175641));
#35333=CARTESIAN_POINT('Ctrl Pts',(-0.288111383720094,-0.959382686643452,
-0.0509606390459395));
#35334=CARTESIAN_POINT('Ctrl Pts',(-0.260526571632154,-0.932962863692293,
-0.418764773197866));
#35335=CARTESIAN_POINT('Ctrl Pts',(-0.209118231971798,-0.457137824406994,
-1.03650380031556));
#35336=CARTESIAN_POINT('Ctrl Pts',(-0.137647649254552,0.62339432936104,
-0.945744416684868));
#35337=CARTESIAN_POINT('Ctrl Pts',(-0.0679415719306187,1.11977874493364,
-0.0128664266509041));
#35338=CARTESIAN_POINT('Ctrl Pts',(-0.0220590221791022,0.806106298516984,
0.59564865151797));
#35339=CARTESIAN_POINT('Ctrl Pts',(-1.14112278654099E-15,0.570663374910285,
0.771750967939217));
#35340=CARTESIAN_POINT('',(0.,0.913908649078052,-0.288121577880467));
#35341=CARTESIAN_POINT('Origin',(0.,0.,0.));
#35342=CARTESIAN_POINT('Ctrl Pts',(-0.203127331764369,-0.958925693334137,
0.000778823732210361));
#35343=CARTESIAN_POINT('Ctrl Pts',(-0.183065276321077,-0.956734059660944,
-0.267117843441326));
#35344=CARTESIAN_POINT('Ctrl Pts',(-0.13917969330537,-0.700830832226228,
-0.857155041760208));
#35345=CARTESIAN_POINT('Ctrl Pts',(-0.0714705827172459,0.300862454100803,
-1.09171050239691));
#35346=CARTESIAN_POINT('Ctrl Pts',(-0.0238235275724158,0.818068118928352,
-0.592123416550042));
#35347=CARTESIAN_POINT('Ctrl Pts',(0.,0.913908649078056,-0.288121577880454));
#35348=CARTESIAN_POINT('Origin',(-8.61687266823562,0.,0.));
#35349=CARTESIAN_POINT('',(-0.741872668235614,-0.956728983665432,-0.000237929659179223));
#35350=CARTESIAN_POINT('',(-0.653127331764369,-0.959131267467959,-0.000696535169553286));
#35351=CARTESIAN_POINT('',(-8.61687266823562,-0.95825,-1.32069628103871E-13));
#35352=CARTESIAN_POINT('Ctrl Pts',(-0.741872668235614,-0.956728983665433,
-0.000237929659179185));
#35353=CARTESIAN_POINT('Ctrl Pts',(-0.731052549154585,-0.957051776896419,
-0.145545400519289));
#35354=CARTESIAN_POINT('Ctrl Pts',(-0.696408902501142,-0.857684767529791,
-0.610369126283467));
#35355=CARTESIAN_POINT('Ctrl Pts',(-0.637941728275282,-0.135206620182443,
-1.12463688374277));
#35356=CARTESIAN_POINT('Ctrl Pts',(-0.566471145558034,0.87179625879392,
-0.723228026706244));
#35357=CARTESIAN_POINT('Ctrl Pts',(-0.495000562840788,1.08031370561788,
0.340570456675246));
#35358=CARTESIAN_POINT('Ctrl Pts',(-0.42352998012354,0.299404286128507,
1.09246172377618));
#35359=CARTESIAN_POINT('Ctrl Pts',(-0.355820681921817,-0.700244095450074,
0.856828377137249));
#35360=CARTESIAN_POINT('Ctrl Pts',(-0.31193491129251,-0.956624260471124,
0.267085417349426));
#35361=CARTESIAN_POINT('Ctrl Pts',(-0.291872668235618,-0.958947183310973,
-0.000747180795175641));
#35362=CARTESIAN_POINT('Ctrl Pts',(-0.653127331764369,-0.959131267467959,
-0.00069653516955346));
#35363=CARTESIAN_POINT('Ctrl Pts',(-0.649829969327988,-0.959491703395879,
-0.0446960802726476));
#35364=CARTESIAN_POINT('Ctrl Pts',(-0.62270907931919,-0.936746049792099,
-0.406219180022716));
#35365=CARTESIAN_POINT('Ctrl Pts',(-0.571764661737977,-0.477113298122812,
-1.02736478175254));
#35366=CARTESIAN_POINT('Ctrl Pts',(-0.50029407902073,0.604749195542173,
-0.957794082086403));
#35367=CARTESIAN_POINT('Ctrl Pts',(-0.428823496303482,1.1326255269949,-0.0110385894026361));
#35368=CARTESIAN_POINT('Ctrl Pts',(-0.357352913586236,0.623328692801092,
0.945926260653483));
#35369=CARTESIAN_POINT('Ctrl Pts',(-0.285882330868988,-0.457232996199784,
1.03633538397604));
#35370=CARTESIAN_POINT('Ctrl Pts',(-0.234473803595033,-0.932756597386936,
0.418887604268179));
#35371=CARTESIAN_POINT('Ctrl Pts',(-0.206888803893493,-0.959336606812183,
0.0510072686643281));
#35372=CARTESIAN_POINT('Ctrl Pts',(-0.203127331764369,-0.958925693334137,
0.000778823732210361));
#35373=CARTESIAN_POINT('Origin',(-8.61687266823562,0.,0.));
#35374=CARTESIAN_POINT('',(-1.19187266823562,-0.958088840212646,0.000876755735238218));
#35375=CARTESIAN_POINT('',(-1.10312733176437,-0.956784848343336,-0.000335004702462158));
#35376=CARTESIAN_POINT('',(-8.61687266823562,-0.95825,-1.32069628103871E-13));
#35377=CARTESIAN_POINT('Ctrl Pts',(-1.19187266823562,-0.958088840212646,
0.000876755735238132));
#35378=CARTESIAN_POINT('Ctrl Pts',(-1.17399371458908,-0.955922435214412,
-0.238368404924597));
#35379=CARTESIAN_POINT('Ctrl Pts',(-1.13229123337013,-0.744142554039245,
-0.799826227319725));
#35380=CARTESIAN_POINT('Ctrl Pts',(-1.06676522457877,0.1983703394913,-1.11522836645996));
#35381=CARTESIAN_POINT('Ctrl Pts',(-0.995294641861518,1.04470289737796,
-0.437813907286639));
#35382=CARTESIAN_POINT('Ctrl Pts',(-0.923824059144271,0.934198937671177,
0.640591100675686));
#35383=CARTESIAN_POINT('Ctrl Pts',(-0.852353476427024,-0.0319309011644629,
1.13228350740848));
#35384=CARTESIAN_POINT('Ctrl Pts',(-0.791703012790804,-0.82697889907382,
0.66948777117457));
#35385=CARTESIAN_POINT('Ctrl Pts',(-0.754876076727001,-0.956341057043799,
0.174389760322289));
#35386=CARTESIAN_POINT('Ctrl Pts',(-0.741872668235614,-0.956728983665433,
-0.000237929659179185));
#35387=CARTESIAN_POINT('Ctrl Pts',(-1.10312733176437,-0.956784848343336,
-0.000335004702462244));
#35388=CARTESIAN_POINT('Ctrl Pts',(-1.09277113476248,-0.957221115285983,
-0.139392137331314));
#35389=CARTESIAN_POINT('Ctrl Pts',(-1.05859141018818,-0.863731290477847,
-0.597779280961512));
#35390=CARTESIAN_POINT('Ctrl Pts',(-1.00058815804146,-0.157032780474456,
-1.12179595235208));
#35391=CARTESIAN_POINT('Ctrl Pts',(-0.929117575324211,0.857575021859809,
-0.740034212889895));
#35392=CARTESIAN_POINT('Ctrl Pts',(-0.857646992606967,1.0867335802145,0.31951868111913));
#35393=CARTESIAN_POINT('Ctrl Pts',(-0.786176409889718,0.320564368022132,
1.08642872230062));
#35394=CARTESIAN_POINT('Ctrl Pts',(-0.718003189608853,-0.690321369002484,
0.868807863254718));
#35395=CARTESIAN_POINT('Ctrl Pts',(-0.673653496900403,-0.956887544637908,
0.2732017535753));
#35396=CARTESIAN_POINT('Ctrl Pts',(-0.653127331764369,-0.959131267467959,
-0.00069653516955346));
#35397=CARTESIAN_POINT('Origin',(-8.61687266823562,0.,0.));
#35398=CARTESIAN_POINT('',(-1.64187266823562,-0.959728790079239,-0.000272255018208681));
#35399=CARTESIAN_POINT('',(-1.55312733176437,-0.957905508838967,0.000864921553367683));
#35400=CARTESIAN_POINT('',(-8.61687266823562,-0.95825,-1.32069628103871E-13));
#35401=CARTESIAN_POINT('Ctrl Pts',(-1.64187266823562,-0.959728790079238,
-0.000272255018208569));
#35402=CARTESIAN_POINT('Ctrl Pts',(-1.64075840759599,-0.959784665653602,
-0.0151165166273389));
#35403=CARTESIAN_POINT('Ctrl Pts',(-1.61582061938395,-0.95274448746835,
-0.347285402846716));
#35404=CARTESIAN_POINT('Ctrl Pts',(-1.5670593035995,-0.568921139707624,
-0.979496698268463));
#35405=CARTESIAN_POINT('Ctrl Pts',(-1.49558872088225,0.514728551628869,
-1.00902902087099));
#35406=CARTESIAN_POINT('Ctrl Pts',(-1.424118138165,1.12694188770285,-0.114398565074092));
#35407=CARTESIAN_POINT('Ctrl Pts',(-1.35264755544776,0.706996853826318,
0.885008749153142));
#35408=CARTESIAN_POINT('Ctrl Pts',(-1.28117697273051,-0.360481749440169,
1.07384261429556));
#35409=CARTESIAN_POINT('Ctrl Pts',(-1.22758534365979,-0.91335198538869,
0.477949908633713));
#35410=CARTESIAN_POINT('Ctrl Pts',(-1.1978172421615,-0.958809148286597,
0.0804233876057907));
#35411=CARTESIAN_POINT('Ctrl Pts',(-1.19187266823562,-0.958088840212646,
0.000876755735238132));
#35412=CARTESIAN_POINT('Ctrl Pts',(-1.55312733176437,-0.957905508838967,
0.000864921553367691));
#35413=CARTESIAN_POINT('Ctrl Pts',(-1.53571230019698,-0.955856605455542,
-0.232285840518138));
#35414=CARTESIAN_POINT('Ctrl Pts',(-1.49447374105717,-0.752915558634865,
-0.787577677013262));
#35415=CARTESIAN_POINT('Ctrl Pts',(-1.42941165434494,0.176662356954578,
-1.11887237535459));
#35416=CARTESIAN_POINT('Ctrl Pts',(-1.3579410716277,1.03599816963305,-0.458031427443242));
#35417=CARTESIAN_POINT('Ctrl Pts',(-1.28647048891045,0.946470301531875,
0.622317346917095));
#35418=CARTESIAN_POINT('Ctrl Pts',(-1.2149999061932,-0.00992315233657026,
1.13268996675844));
#35419=CARTESIAN_POINT('Ctrl Pts',(-1.15388552047784,-0.819962267279029,
0.682009929435178));
#35420=CARTESIAN_POINT('Ctrl Pts',(-1.1165946623349,-0.956217521250915,
0.180496662845114));
#35421=CARTESIAN_POINT('Ctrl Pts',(-1.10312733176437,-0.956784848343336,
-0.000335004702462244));
#35422=CARTESIAN_POINT('Origin',(-8.61687266823562,0.,0.));
#35423=CARTESIAN_POINT('',(-2.09187266823562,-0.957282800009966,-0.000711420515223326));
#35424=CARTESIAN_POINT('',(-2.00312733176437,-0.959789721040338,-0.000160985410693898));
#35425=CARTESIAN_POINT('',(-8.61687266823562,-0.95825,-1.32069628103871E-13));
#35426=CARTESIAN_POINT('Ctrl Pts',(-2.09187266823562,-0.957282800009966,
-0.000711420515223399));
#35427=CARTESIAN_POINT('Ctrl Pts',(-2.08369957303049,-0.958037494378474,
-0.110312090770477));
#35428=CARTESIAN_POINT('Ctrl Pts',(-2.05170295025294,-0.890024371399682,
-0.538476540815407));
#35429=CARTESIAN_POINT('Ctrl Pts',(-1.99588279990298,-0.258816672158623,
-1.10276877747064));
#35430=CARTESIAN_POINT('Ctrl Pts',(-1.92441221718573,0.786412695849304,
-0.815254633948207));
#35431=CARTESIAN_POINT('Ctrl Pts',(-1.85294163446849,1.11137205677529,0.218945650531032));
#35432=CARTESIAN_POINT('Ctrl Pts',(-1.78147105175124,0.418433355264041,
1.05261511171313));
#35433=CARTESIAN_POINT('Ctrl Pts',(-1.71111472967362,-0.640967447381487,
0.924234803949312));
#35434=CARTESIAN_POINT('Ctrl Pts',(-1.66458193516841,-0.958590014026201,
0.302262257387501));
#35435=CARTESIAN_POINT('Ctrl Pts',(-1.64187266823562,-0.959728790079238,
-0.000272255018208569));
#35436=CARTESIAN_POINT('Ctrl Pts',(-2.00312733176437,-0.959789721040338,
-0.000160985410693976));
#35437=CARTESIAN_POINT('Ctrl Pts',(-2.00247699320389,-0.959809874352138,
-0.00882337026222604));
#35438=CARTESIAN_POINT('Ctrl Pts',(-1.97800312707099,-0.955778669076828,
-0.334791339982387));
#35439=CARTESIAN_POINT('Ctrl Pts',(-1.92970573336567,-0.587846795790038,
-0.968256742613268));
#35440=CARTESIAN_POINT('Ctrl Pts',(-1.85823515064843,0.4950244060751,-1.01884042543795));
#35441=CARTESIAN_POINT('Ctrl Pts',(-1.78676456793118,1.12450614210672,-0.13627513368518));
#35442=CARTESIAN_POINT('Ctrl Pts',(-1.71529398521393,0.724060395961153,
0.871103620044959));
#35443=CARTESIAN_POINT('Ctrl Pts',(-1.64382340249668,-0.339547310642638,
1.08064452961661));
#35444=CARTESIAN_POINT('Ctrl Pts',(-1.58976785134683,-0.908777537601796,
0.490543016397207));
#35445=CARTESIAN_POINT('Ctrl Pts',(-1.55953582776939,-0.958659477564004,
0.0866612476479209));
#35446=CARTESIAN_POINT('Ctrl Pts',(-1.55312733176437,-0.957905508838967,
0.000864921553367691));
#35447=CARTESIAN_POINT('Origin',(-8.61687266823562,0.,0.));
#35448=CARTESIAN_POINT('',(-2.54187266823562,-0.957160045438329,0.000652648723329974));
#35449=CARTESIAN_POINT('',(-2.45312733176437,-0.957431559463739,-0.000767278543180316));
#35450=CARTESIAN_POINT('',(-8.61687266823562,-0.95825,-1.32069628103871E-13));
#35451=CARTESIAN_POINT('Ctrl Pts',(-2.54187266823562,-0.957160045438329,
0.000652648723330016));
#35452=CARTESIAN_POINT('Ctrl Pts',(-2.52664073846498,-0.955880301498824,
-0.203672381995242));
#35453=CARTESIAN_POINT('Ctrl Pts',(-2.48758528112193,-0.791644135614284,
-0.729450334203188));
#35454=CARTESIAN_POINT('Ctrl Pts',(-2.42470629620646,0.0737508650376029,
-1.13032997672338));
#35455=CARTESIAN_POINT('Ctrl Pts',(-2.35323571348922,0.989842956438803,
-0.550723131856308));
#35456=CARTESIAN_POINT('Ctrl Pts',(-2.28176513077197,0.999344656976215,
0.533287261191272));
#35457=CARTESIAN_POINT('Ctrl Pts',(-2.21029454805472,0.0935534241382057,
1.12886350069563));
#35458=CARTESIAN_POINT('Ctrl Pts',(-2.1469970605426,-0.784541427588874,
0.740648467365689));
#35459=CARTESIAN_POINT('Ctrl Pts',(-2.1075231006029,-0.955837656783825,
0.209159850305441));
#35460=CARTESIAN_POINT('Ctrl Pts',(-2.09187266823562,-0.957282800009966,
-0.000711420515223399));
#35461=CARTESIAN_POINT('Ctrl Pts',(-2.45312733176437,-0.957431559463739,
-0.000767278543180386));
#35462=CARTESIAN_POINT('Ctrl Pts',(-2.44541815863838,-0.958207306895283,
-0.104106321084798));
#35463=CARTESIAN_POINT('Ctrl Pts',(-2.41388545793998,-0.895165853018041,
-0.525871241247474));
#35464=CARTESIAN_POINT('Ctrl Pts',(-2.35852922966916,-0.280196248383438,
-1.09753133781927));
#35465=CARTESIAN_POINT('Ctrl Pts',(-2.28705864695191,0.770422572284684,
-0.830381861084687));
#35466=CARTESIAN_POINT('Ctrl Pts',(-2.21558806423466,1.11541663057547,0.197308680388403));
#35467=CARTESIAN_POINT('Ctrl Pts',(-2.14411748151742,0.438808229068046,
1.04428555155484));
#35468=CARTESIAN_POINT('Ctrl Pts',(-2.07329723736065,-0.62988784727845,
0.935804606318756));
#35469=CARTESIAN_POINT('Ctrl Pts',(-2.0263005207763,-0.959071608149721,
0.308501446215017));
#35470=CARTESIAN_POINT('Ctrl Pts',(-2.00312733176437,-0.959789721040338,
-0.000160985410693976));
#35471=CARTESIAN_POINT('Origin',(-8.61687266823562,0.,0.));
#35472=CARTESIAN_POINT('',(-2.99187266823562,-0.959650450245746,0.000368126650595699));
#35473=CARTESIAN_POINT('',(-2.90312733176437,-0.957038006623854,0.000579103131620948));
#35474=CARTESIAN_POINT('',(-8.61687266823562,-0.95825,-1.32069628103871E-13));
#35475=CARTESIAN_POINT('Ctrl Pts',(-2.99187266823562,-0.959650450245746,
0.000368126650595773));
#35476=CARTESIAN_POINT('Ctrl Pts',(-2.96958190389948,-0.958193208886187,
-0.296655628075332));
#35477=CARTESIAN_POINT('Ctrl Pts',(-2.92346761199092,-0.650782839392722,
-0.913731080697807));
#35478=CARTESIAN_POINT('Ctrl Pts',(-2.85352979250995,0.399917459173323,
-1.05978822045819));
#35479=CARTESIAN_POINT('Ctrl Pts',(-2.78205920979269,1.10736333094316,-0.238393581406989));
#35480=CARTESIAN_POINT('Ctrl Pts',(-2.71058862707545,0.800582704964894,
0.801344107662086));
#35481=CARTESIAN_POINT('Ctrl Pts',(-2.6391180443582,-0.239446142554869,
1.10713621166916));
#35482=CARTESIAN_POINT('Ctrl Pts',(-2.58287939141159,-0.885254315562734,
0.549848221345033));
#35483=CARTESIAN_POINT('Ctrl Pts',(-2.5504642660374,-0.957881887344315,
0.115902555413056));
#35484=CARTESIAN_POINT('Ctrl Pts',(-2.54187266823562,-0.957160045438329,
0.000652648723330016));
#35485=CARTESIAN_POINT('Ctrl Pts',(-2.90312733176437,-0.957038006623854,
0.000579103131620913));
#35486=CARTESIAN_POINT('Ctrl Pts',(-2.88835932407288,-0.955945717746202,
-0.197586125297776));
#35487=CARTESIAN_POINT('Ctrl Pts',(-2.84976778880897,-0.799342738306937,
-0.71701096012948));
#35488=CARTESIAN_POINT('Ctrl Pts',(-2.78735272597264,0.051772932289347,
-1.13154961826182));
#35489=CARTESIAN_POINT('Ctrl Pts',(-2.71588214325539,0.978954661287059,
-0.569853267298351));
#35490=CARTESIAN_POINT('Ctrl Pts',(-2.64441156053815,1.00951851444678,0.513767791999302));
#35491=CARTESIAN_POINT('Ctrl Pts',(-2.5729409778209,0.115471267790065,1.12683244602779));
#35492=CARTESIAN_POINT('Ctrl Pts',(-2.50917956822964,-0.776491202911252,
0.753033696487916));
#35493=CARTESIAN_POINT('Ctrl Pts',(-2.4692416862108,-0.955810027703003,
0.215240577611453));
#35494=CARTESIAN_POINT('Ctrl Pts',(-2.45312733176437,-0.957431559463739,
-0.000767278543180386));
#35495=CARTESIAN_POINT('Origin',(-8.61687266823562,0.,0.));
#35496=CARTESIAN_POINT('',(-3.44187266823562,-0.958257665410638,-0.000876459478439951));
#35497=CARTESIAN_POINT('',(-3.35312733176437,-0.959540833023362,0.000467762790667282));
#35498=CARTESIAN_POINT('',(-8.61687266823562,-0.95825,-1.32069628103871E-13));
#35499=CARTESIAN_POINT('Ctrl Pts',(-3.44187266823562,-0.958257665410638,
-0.00087645947844002));
#35500=CARTESIAN_POINT('Ctrl Pts',(-3.43634659690639,-0.958937642601644,
-0.0747896866542515));
#35501=CARTESIAN_POINT('Ctrl Pts',(-3.40699699800474,-0.917354581093434,
-0.466594412511799));
#35502=CARTESIAN_POINT('Ctrl Pts',(-3.35382387153068,-0.379250074662353,
-1.06735862166481));
#35503=CARTESIAN_POINT('Ctrl Pts',(-3.28235328881343,0.69137464498329,-0.897265928611934));
#35504=CARTESIAN_POINT('Ctrl Pts',(-3.21088270609618,1.12877405797548,0.0946264889719359));
#35505=CARTESIAN_POINT('Ctrl Pts',(-3.13941212337894,0.532337034832168,
0.999851152782103));
#35506=CARTESIAN_POINT('Ctrl Pts',(-3.06794154066169,-0.551663836031854,
0.989318987176647));
#35507=CARTESIAN_POINT('Ctrl Pts',(-3.01876172228058,-0.949899269571083,
0.358565498699607));
#35508=CARTESIAN_POINT('Ctrl Pts',(-2.99340543147189,-0.959750653448679,
0.0207921500119563));
#35509=CARTESIAN_POINT('Ctrl Pts',(-2.99187266823562,-0.959650450245746,
0.000368126650595773));
#35510=CARTESIAN_POINT('Ctrl Pts',(-3.35312733176437,-0.959540833023362,
0.000467762790667295));
#35511=CARTESIAN_POINT('Ctrl Pts',(-3.33130048950737,-0.957793875791413,
-0.290462270881725));
#35512=CARTESIAN_POINT('Ctrl Pts',(-3.28565011967796,-0.661465590816773,
-0.902016944463262));
#35513=CARTESIAN_POINT('Ctrl Pts',(-3.21617622227613,0.379248666114025,
-1.0673590887593));
#35514=CARTESIAN_POINT('Ctrl Pts',(-3.14470563955887,1.10252187493073,-0.259866293323276));
#35515=CARTESIAN_POINT('Ctrl Pts',(-3.07323505684163,0.816002842433735,
0.785636262049064));
#35516=CARTESIAN_POINT('Ctrl Pts',(-3.00176447412438,-0.217887610001112,
1.11157994067649));
#35517=CARTESIAN_POINT('Ctrl Pts',(-2.94506189909863,-0.879818475118968,
0.562453432935334));
#35518=CARTESIAN_POINT('Ctrl Pts',(-2.91218285164529,-0.957707781711591,
0.122091036442916));
#35519=CARTESIAN_POINT('Ctrl Pts',(-2.90312733176437,-0.957038006623854,
0.000579103131620913));
#35520=CARTESIAN_POINT('Origin',(-8.61687266823562,0.,0.));
#35521=CARTESIAN_POINT('',(-3.89187266823562,-0.956695459968737,0.000147939248303057));
#35522=CARTESIAN_POINT('',(-3.80312733176437,-0.958446399572106,-0.000863762433619825));
#35523=CARTESIAN_POINT('',(-8.61687266823562,-0.95825,-1.32069628103871E-13));
#35524=CARTESIAN_POINT('Ctrl Pts',(-3.89187266823562,-0.956695459968737,
0.000147939248303051));
#35525=CARTESIAN_POINT('Ctrl Pts',(-3.87928776234088,-0.956462580794984,
-0.168874488277431));
#35526=CARTESIAN_POINT('Ctrl Pts',(-3.84287932887373,-0.833157873073766,
-0.658177943823049));
#35527=CARTESIAN_POINT('Ctrl Pts',(-3.78264736783416,-0.0517744158194337,
-1.13154958187441));
#35528=CARTESIAN_POINT('Ctrl Pts',(-3.71117678511691,0.922826436408769,
-0.65686864336692));
#35529=CARTESIAN_POINT('Ctrl Pts',(-3.63970620239967,1.05221686991099,0.419433791018696));
#35530=CARTESIAN_POINT('Ctrl Pts',(-3.56823561968242,0.217889071988309,
1.11157968615915));
#35531=CARTESIAN_POINT('Ctrl Pts',(-3.50229110829441,-0.7360618847371,0.810839058251395));
#35532=CARTESIAN_POINT('Ctrl Pts',(-3.4601701244788,-0.956006182909324,
0.243858716647063));
#35533=CARTESIAN_POINT('Ctrl Pts',(-3.44187266823562,-0.958257665410638,
-0.00087645947844002));
#35534=CARTESIAN_POINT('Ctrl Pts',(-3.80312733176437,-0.958446399572106,
-0.000863762433619868));
#35535=CARTESIAN_POINT('Ctrl Pts',(-3.79806518251428,-0.959072080853087,
-0.0685377004959773));
#35536=CARTESIAN_POINT('Ctrl Pts',(-3.76917950569178,-0.921655890668159,
-0.454012480968252));
#35537=CARTESIAN_POINT('Ctrl Pts',(-3.71647030129686,-0.399918836166434,
-1.05978766721718));
#35538=CARTESIAN_POINT('Ctrl Pts',(-3.6449997185796,0.673808865727154,-0.910530937186564));
#35539=CARTESIAN_POINT('Ctrl Pts',(-3.57352913586236,1.13039963799526,0.072674847963582));
#35540=CARTESIAN_POINT('Ctrl Pts',(-3.50205855314511,0.551665116510674,
0.989318237136875));
#35541=CARTESIAN_POINT('Ctrl Pts',(-3.43058797042786,-0.532335710452797,
0.999851822263215));
#35542=CARTESIAN_POINT('Ctrl Pts',(-3.38094422996762,-0.946623962906586,
0.371079864210543));
#35543=CARTESIAN_POINT('Ctrl Pts',(-3.35512401707979,-0.959700641932531,
0.0270815862291171));
#35544=CARTESIAN_POINT('Ctrl Pts',(-3.35312733176437,-0.959540833023362,
0.000467762790667295));
#35545=CARTESIAN_POINT('Origin',(-8.61687266823562,0.,0.));
#35546=CARTESIAN_POINT('',(-4.34187266823562,-0.958801047132561,0.000803658998405769));
#35547=CARTESIAN_POINT('',(-4.25312733176437,-0.956676639742279,4.61738887314045E-5));
#35548=CARTESIAN_POINT('',(-8.61687266823562,-0.95825,-1.32069628103871E-13));
#35549=CARTESIAN_POINT('Ctrl Pts',(-4.34187266823562,-0.958801047132561,
0.000803658998405725));
#35550=CARTESIAN_POINT('Ctrl Pts',(-4.32222892777538,-0.956446580846668,
-0.261555840640749));
#35551=CARTESIAN_POINT('Ctrl Pts',(-4.27876165974272,-0.708980756137565,
-0.846004557974328));
#35552=CARTESIAN_POINT('Ctrl Pts',(-4.21147086413764,0.280194818630884,
-1.09753173529789));
#35553=CARTESIAN_POINT('Ctrl Pts',(-4.1400002814204,1.07418480140191,-0.359460788975286));
#35554=CARTESIAN_POINT('Ctrl Pts',(-4.06852969870314,0.884336274609667,
0.707837834382355));
#35555=CARTESIAN_POINT('Ctrl Pts',(-3.99705911598591,-0.115469795083229,
1.12683262856426));
#35556=CARTESIAN_POINT('Ctrl Pts',(-3.93817343916339,-0.85208931007107,
0.621720486442062));
#35557=CARTESIAN_POINT('Ctrl Pts',(-3.9031112899133,-0.956903426635498,
0.151089005784113));
#35558=CARTESIAN_POINT('Ctrl Pts',(-3.89187266823562,-0.956695459968737,
0.000147939248303051));
#35559=CARTESIAN_POINT('Ctrl Pts',(-4.25312733176437,-0.956676639742279,
4.61738887314392E-5));
#35560=CARTESIAN_POINT('Ctrl Pts',(-4.24100634794878,-0.956606710883735,
-0.162753489137796));
#35561=CARTESIAN_POINT('Ctrl Pts',(-4.20506183656076,-0.839843493636197,
-0.645626437601176));
#35562=CARTESIAN_POINT('Ctrl Pts',(-4.14529379760033,-0.0737523434839011,
-1.1303298487331));
#35563=CARTESIAN_POINT('Ctrl Pts',(-4.07382321488309,0.909888230063614,
-0.674676503146548));
#35564=CARTESIAN_POINT('Ctrl Pts',(-4.00235263216584,1.06016839954784,0.398908435241142));
#35565=CARTESIAN_POINT('Ctrl Pts',(-3.93088204944859,0.239447586020594,
1.1071358672969));
#35566=CARTESIAN_POINT('Ctrl Pts',(-3.86447361598144,-0.726917995153459,
0.823003811913429));
#35567=CARTESIAN_POINT('Ctrl Pts',(-3.8218887100867,-0.956127494569163,
0.249949931873536));
#35568=CARTESIAN_POINT('Ctrl Pts',(-3.80312733176437,-0.958446399572106,
-0.000863762433619868));
#35569=CARTESIAN_POINT('Origin',(-8.61687266823562,0.,0.));
#35570=CARTESIAN_POINT('',(-4.79187266823562,-0.959278083226344,-0.00063277652707348));
#35571=CARTESIAN_POINT('',(-4.70312733176437,-0.958616057498963,0.000841104330781481));
#35572=CARTESIAN_POINT('',(-8.61687266823562,-0.95825,-1.32069628103871E-13));
#35573=CARTESIAN_POINT('Ctrl Pts',(-4.79187266823562,-0.959278083226344,
-0.000632776527073604));
#35574=CARTESIAN_POINT('Ctrl Pts',(-4.78899362078229,-0.959570967253412,
-0.0390352664624121));
#35575=CARTESIAN_POINT('Ctrl Pts',(-4.76229104575654,-0.940036834855403,
-0.394909991490227));
#35576=CARTESIAN_POINT('Ctrl Pts',(-4.71176494315838,-0.495025754436958,
-1.01883980527742));
#35577=CARTESIAN_POINT('Ctrl Pts',(-4.64029436044113,0.587845543979899,
-0.968257539498959));
#35578=CARTESIAN_POINT('Ctrl Pts',(-4.56882377772388,1.13231313096107,-0.0308548185336372));
#35579=CARTESIAN_POINT('Ctrl Pts',(-4.49735319500663,0.639702869075108,
0.934807619604525));
#35580=CARTESIAN_POINT('Ctrl Pts',(-4.42588261228939,-0.438806873470812,
1.0442861553082));
#35581=CARTESIAN_POINT('Ctrl Pts',(-4.37405577003238,-0.92944979296497,
0.430102104777608));
#35582=CARTESIAN_POINT('Ctrl Pts',(-4.34605245534779,-0.959302029512049,
0.0566284067121712));
#35583=CARTESIAN_POINT('Ctrl Pts',(-4.34187266823562,-0.958801047132561,
0.000803658998405725));
#35584=CARTESIAN_POINT('Ctrl Pts',(-4.70312733176437,-0.958616057498963,
0.000841104330781481));
#35585=CARTESIAN_POINT('Ctrl Pts',(-4.68394751338327,-0.956263924788962,
-0.255449887934941));
#35586=CARTESIAN_POINT('Ctrl Pts',(-4.64094416742975,-0.718501334310948,
-0.833934531383708));
#35587=CARTESIAN_POINT('Ctrl Pts',(-4.57411729390382,0.258815220585386,
-1.10276908584694));
#35588=CARTESIAN_POINT('Ctrl Pts',(-4.50264671118657,1.06699709340334,-0.380265930337164));
#35589=CARTESIAN_POINT('Ctrl Pts',(-4.43117612846933,0.897923629232473,
0.690520188823135));
#35590=CARTESIAN_POINT('Ctrl Pts',(-4.35970554575208,-0.093551942967458,
1.12886359188051));
#35591=CARTESIAN_POINT('Ctrl Pts',(-4.30035594685043,-0.845727021412224,
0.634294523148357));
#35592=CARTESIAN_POINT('Ctrl Pts',(-4.26482987552119,-0.956744154519911,
0.157225674261628));
#35593=CARTESIAN_POINT('Ctrl Pts',(-4.25312733176437,-0.956676639742279,
4.61738887314392E-5));
#35594=CARTESIAN_POINT('Origin',(-8.61687266823562,0.,0.));
#35595=CARTESIAN_POINT('',(-5.24187266823562,-0.956851161348753,-0.000418646029398152));
#35596=CARTESIAN_POINT('',(-5.15312733176438,-0.959424157494653,-0.000550396959753813));
#35597=CARTESIAN_POINT('',(-8.61687266823562,-0.95825,-1.32069628103871E-13));
#35598=CARTESIAN_POINT('Ctrl Pts',(-5.24187266823562,-0.956851161348753,
-0.000418646029398334));
#35599=CARTESIAN_POINT('Ctrl Pts',(-5.23193478621678,-0.957376403620873,
-0.133835808799005));
#35600=CARTESIAN_POINT('Ctrl Pts',(-5.19817337662553,-0.869043093986714,
-0.586421640241982));
#35601=CARTESIAN_POINT('Ctrl Pts',(-5.14058843946185,-0.176663834249519,
-1.11887217144864));
#35602=CARTESIAN_POINT('Ctrl Pts',(-5.06911785674461,0.844476313709149,
-0.754946886845504));
#35603=CARTESIAN_POINT('Ctrl Pts',(-4.99764727402736,1.09216638421668,0.30042908574342));
#35604=CARTESIAN_POINT('Ctrl Pts',(-4.92617669131012,0.339548736498745,
1.08064411436687));
#35605=CARTESIAN_POINT('Ctrl Pts',(-4.8575851560462,-0.681213984298933,
0.879545467471477));
#35606=CARTESIAN_POINT('Ctrl Pts',(-4.8128171483547,-0.957147411960396,
0.278737466586754));
#35607=CARTESIAN_POINT('Ctrl Pts',(-4.79187266823562,-0.959278083226344,
-0.000632776527073604));
#35608=CARTESIAN_POINT('Ctrl Pts',(-5.15312733176438,-0.959424157494653,
-0.00055039695975393));
#35609=CARTESIAN_POINT('Ctrl Pts',(-5.15071220639018,-0.95964469725191,
-0.0327519345529813));
#35610=CARTESIAN_POINT('Ctrl Pts',(-5.12447355344357,-0.943559089128387,
-0.382376225977263));
#35611=CARTESIAN_POINT('Ctrl Pts',(-5.07441137292454,-0.514729859854887,
-1.00902831797734));
#35612=CARTESIAN_POINT('Ctrl Pts',(-5.00294079020731,0.56891984144925,-0.979497416592661));
#35613=CARTESIAN_POINT('Ctrl Pts',(-4.93147020749005,1.13149975276759,-0.0528515334991769));
#35614=CARTESIAN_POINT('Ctrl Pts',(-4.85999962477281,0.657746782740738,
0.92220070749299));
#35615=CARTESIAN_POINT('Ctrl Pts',(-4.78852904205556,-0.418431965008117,
1.05261563059162));
#35616=CARTESIAN_POINT('Ctrl Pts',(-4.73623827771942,-0.925414685010962,
0.442670069694638));
#35617=CARTESIAN_POINT('Ctrl Pts',(-4.70777104095569,-0.959185542572679,
0.0628928304100949));
#35618=CARTESIAN_POINT('Ctrl Pts',(-4.70312733176437,-0.958616057498963,
0.000841104330781481));
#35619=CARTESIAN_POINT('Origin',(-8.61687266823562,0.,0.));
#35620=CARTESIAN_POINT('',(-5.69187266823562,-0.957745541375101,0.000843587520472362));
#35621=CARTESIAN_POINT('',(-5.60312733176437,-0.956941681982296,-0.000506047312858471));
#35622=CARTESIAN_POINT('',(-8.61687266823562,-0.95825,-1.32069628103871E-13));
#35623=CARTESIAN_POINT('Ctrl Pts',(-5.69187266823562,-0.957745541375101,
0.00084358752047234));
#35624=CARTESIAN_POINT('Ctrl Pts',(-5.67487595165128,-0.955820359152125,
-0.226803304052992));
#35625=CARTESIAN_POINT('Ctrl Pts',(-5.63405570749452,-0.760661038176944,
-0.776499075945558));
#35626=CARTESIAN_POINT('Ctrl Pts',(-5.56941193576534,0.157030992812372,
-1.1217960214248));
#35627=CARTESIAN_POINT('Ctrl Pts',(-5.49794135304809,1.02781377622821,-0.476113313998863));
#35628=CARTESIAN_POINT('Ctrl Pts',(-5.42647077033084,0.957228954744552,
0.605638319931491));
#35629=CARTESIAN_POINT('Ctrl Pts',(-5.3550001876136,0.00992468338927851,
1.13268996068449));
#35630=CARTESIAN_POINT('Ctrl Pts',(-5.29346748691519,-0.813484292874832,
0.69328502015914));
#35631=CARTESIAN_POINT('Ctrl Pts',(-5.2557583137892,-0.956117269760326,
0.185997677838279));
#35632=CARTESIAN_POINT('Ctrl Pts',(-5.24187266823562,-0.956851161348753,
-0.000418646029398334));
#35633=CARTESIAN_POINT('Ctrl Pts',(-5.60312733176437,-0.956941681982296,
-0.000506047312858627));
#35634=CARTESIAN_POINT('Ctrl Pts',(-5.59365337182468,-0.957550312161305,
-0.127664896619225));
#35635=CARTESIAN_POINT('Ctrl Pts',(-5.56035588431256,-0.874780422660147,
-0.573821257585252));
#35636=CARTESIAN_POINT('Ctrl Pts',(-5.50323486922804,-0.198371837060489,
-1.11522804366184));
#35637=CARTESIAN_POINT('Ctrl Pts',(-5.43176428651079,0.829647095487569,
-0.771213765472918));
#35638=CARTESIAN_POINT('Ctrl Pts',(-5.36029370379354,1.09779793008511,0.279149923530103));
#35639=CARTESIAN_POINT('Ctrl Pts',(-5.28882312107629,0.360483152130068,
1.07384210763829));
#35640=CARTESIAN_POINT('Ctrl Pts',(-5.21976766373324,-0.670923561447508,
0.89139065675279));
#35641=CARTESIAN_POINT('Ctrl Pts',(-5.1745357339626,-0.957469226345113,
0.28489377731112));
#35642=CARTESIAN_POINT('Ctrl Pts',(-5.15312733176438,-0.959424157494653,
-0.00055039695975393));
#35643=CARTESIAN_POINT('Origin',(-8.61687266823562,0.,0.));
#35644=CARTESIAN_POINT('',(-6.14187266823562,-0.959818611724535,-5.7784059915537E-5));
#35645=CARTESIAN_POINT('',(-6.05312733176438,-0.957575902522396,0.000808576896546773));
#35646=CARTESIAN_POINT('',(-8.61687266823562,-0.95825,-1.32069628103871E-13));
#35647=CARTESIAN_POINT('Ctrl Pts',(-6.14187266823562,-0.959818611724535,
-5.77840599154589E-5));
#35648=CARTESIAN_POINT('Ctrl Pts',(-6.14164064465819,-0.95982130723207,
-0.0031480436667598));
#35649=CARTESIAN_POINT('Ctrl Pts',(-6.11758509350833,-0.958407877072966,
-0.323534921547347));
#35650=CARTESIAN_POINT('Ctrl Pts',(-6.06970601478608,-0.604721823700482,
-0.957808206827138));
#35651=CARTESIAN_POINT('Ctrl Pts',(-5.99823543206882,0.47709687534022,-1.02735759037585));
#35652=CARTESIAN_POINT('Ctrl Pts',(-5.92676484935158,1.12194581094373,-0.155957185437944));
#35653=CARTESIAN_POINT('Ctrl Pts',(-5.85529426663432,0.739212255050342,
0.858283337941351));
#35654=CARTESIAN_POINT('Ctrl Pts',(-5.78382368391709,-0.320560747180587,
1.08642802515142));
#35655=CARTESIAN_POINT('Ctrl Pts',(-5.72934981778418,-0.904527421769531,
0.501902134781091));
#35656=CARTESIAN_POINT('Ctrl Pts',(-5.69869947922369,-0.958518799850562,
0.0922790299532361));
#35657=CARTESIAN_POINT('Ctrl Pts',(-5.69187266823562,-0.957745541375101,
0.00084358752047234));
#35658=CARTESIAN_POINT('Ctrl Pts',(-6.05312733176438,-0.957575902522396,
0.000808576896546643));
#35659=CARTESIAN_POINT('Ctrl Pts',(-6.03659453725917,-0.95580418331262,
-0.220724011270484));
#35660=CARTESIAN_POINT('Ctrl Pts',(-5.99623821518156,-0.769069431346248,
-0.764177221634974));
#35661=CARTESIAN_POINT('Ctrl Pts',(-5.93205836553151,0.135203161210182,
-1.12463553224998));
#35662=CARTESIAN_POINT('Ctrl Pts',(-5.86058778281427,1.01836809138401,-0.495995368476964));
#35663=CARTESIAN_POINT('Ctrl Pts',(-5.78911720009702,0.968816654749839,
0.586923559386877));
#35664=CARTESIAN_POINT('Ctrl Pts',(-5.71764661737977,0.0319326731109062,
1.13228321523766));
#35665=CARTESIAN_POINT('Ctrl Pts',(-5.65564999460223,-0.806130353491351,
0.705769711573949));
#35666=CARTESIAN_POINT('Ctrl Pts',(-5.61747689939709,-0.956019830932409,
0.192092878567596));
#35667=CARTESIAN_POINT('Ctrl Pts',(-5.60312733176437,-0.956941681982296,
-0.000506047312858627));
#35668=CARTESIAN_POINT('Origin',(-8.61687266823562,0.,0.));
#35669=CARTESIAN_POINT('',(-6.59187266823562,-0.957575883836689,-0.000808561082841419));
#35670=CARTESIAN_POINT('',(-6.50312733176438,-0.959818590364428,5.77507014088265E-5));
#35671=CARTESIAN_POINT('',(-8.61687266823562,-0.95825,-1.32069628103871E-13));
#35672=CARTESIAN_POINT('Ctrl Pts',(-6.59187266823562,-0.957575883836689,
-0.000808561082841245));
#35673=CARTESIAN_POINT('Ctrl Pts',(-6.58458181009268,-0.958357188928375,
-0.0985030576430004));
#35674=CARTESIAN_POINT('Ctrl Pts',(-6.55346742437732,-0.899671699226215,
-0.514506640016404));
#35675=CARTESIAN_POINT('Ctrl Pts',(-6.49852951108958,-0.299383568459973,
-1.09245341423609));
#35676=CARTESIAN_POINT('Ctrl Pts',(-6.42705892837228,0.755754835285377,
-0.843753338464662));
#35677=CARTESIAN_POINT('Ctrl Pts',(-6.35558834565508,1.11870256511677,0.177734697675315));
#35678=CARTESIAN_POINT('Ctrl Pts',(-6.28411776293779,0.457038265720188,
1.03643671348781));
#35679=CARTESIAN_POINT('Ctrl Pts',(-6.21287920379801,-0.6197172650586,0.946167455774252));
#35680=CARTESIAN_POINT('Ctrl Pts',(-6.1654641722306,-0.959544540108726,
0.314151110856649));
#35681=CARTESIAN_POINT('Ctrl Pts',(-6.14187266823562,-0.959818611724535,
-5.77840599154589E-5));
#35682=CARTESIAN_POINT('Ctrl Pts',(-6.50312733176438,-0.959818590364428,
5.77507014088167E-5));
#35683=CARTESIAN_POINT('Ctrl Pts',(-6.47953570269367,-0.959544661648279,
-0.314152798513479));
#35684=CARTESIAN_POINT('Ctrl Pts',(-6.43212054605054,-0.619714180231002,
-0.94617051184503));
#35685=CARTESIAN_POINT('Ctrl Pts',(-6.360881861835,0.457043683047776,-1.03643429626688));
#35686=CARTESIAN_POINT('Ctrl Pts',(-6.28941127911776,1.11870346430575,-0.177728822944574));
#35687=CARTESIAN_POINT('Ctrl Pts',(-6.2179406964005,0.755750395960032,0.843757259442018));
#35688=CARTESIAN_POINT('Ctrl Pts',(-6.14647011368326,-0.299389288185346,
1.09245184324826));
#35689=CARTESIAN_POINT('Ctrl Pts',(-6.09153232547121,-0.899672997516219,
0.514503194076797));
#35690=CARTESIAN_POINT('Ctrl Pts',(-6.06041806483159,-0.958357206120191,
0.098501375624914));
#35691=CARTESIAN_POINT('Ctrl Pts',(-6.05312733176438,-0.957575902522396,
0.000808576896546643));
#35692=CARTESIAN_POINT('Origin',(-8.61687266823562,0.,0.));
#35693=CARTESIAN_POINT('',(-7.04187266823562,-0.956941536305503,0.000507261239360324));
#35694=CARTESIAN_POINT('',(-6.95312733176437,-0.957745460096,-0.000843557184232457));
#35695=CARTESIAN_POINT('',(-8.61687266823562,-0.95825,-1.32069628103871E-13));
#35696=CARTESIAN_POINT('Ctrl Pts',(-7.04187266823562,-0.956941536305503,
0.000507261239360299));
#35697=CARTESIAN_POINT('Ctrl Pts',(-7.02752297552718,-0.956019718516196,
-0.19209383932285));
#35698=CARTESIAN_POINT('Ctrl Pts',(-6.98934975524631,-0.806128695492176,
-0.705775048482281));
#35699=CARTESIAN_POINT('Ctrl Pts',(-6.92735300739304,0.0319388218506953,
-1.1322817885948));
#35700=CARTESIAN_POINT('Ctrl Pts',(-6.85588242467578,0.968819643033635,
-0.586919179874541));
#35701=CARTESIAN_POINT('Ctrl Pts',(-6.78441184195855,1.0183655808885,0.496001075865819));
#35702=CARTESIAN_POINT('Ctrl Pts',(-6.71294125924129,0.135197241307266,
1.12463608307476));
#35703=CARTESIAN_POINT('Ctrl Pts',(-6.648761534667,-0.769071682396365,0.764173986137034));
#35704=CARTESIAN_POINT('Ctrl Pts',(-6.60840533766509,-0.955804205036859,
0.220722400710996));
#35705=CARTESIAN_POINT('Ctrl Pts',(-6.59187266823562,-0.957575883836689,
-0.000808561082841245));
#35706=CARTESIAN_POINT('Ctrl Pts',(-6.95312733176437,-0.957745460096,-0.000843557184232414));
#35707=CARTESIAN_POINT('Ctrl Pts',(-6.94630039570057,-0.958518738839012,
-0.0922807305074193));
#35708=CARTESIAN_POINT('Ctrl Pts',(-6.91564993206436,-0.904526183542863,
-0.501905736657279));
#35709=CARTESIAN_POINT('Ctrl Pts',(-6.86117594085573,-0.32055498375887,
-1.08642949326629));
#35710=CARTESIAN_POINT('Ctrl Pts',(-6.78970535813849,0.739216698253442,
-0.858279536751942));
#35711=CARTESIAN_POINT('Ctrl Pts',(-6.71823477542123,1.12194498002037,0.155963109595212));
#35712=CARTESIAN_POINT('Ctrl Pts',(-6.64676419270399,0.477091470497689,
1.02736003461986));
#35713=CARTESIAN_POINT('Ctrl Pts',(-6.57529360998674,-0.604726820287475,
0.957805026523516));
#35714=CARTESIAN_POINT('Ctrl Pts',(-6.5274146563402,-0.958408621577299,
0.323531547364598));
#35715=CARTESIAN_POINT('Ctrl Pts',(-6.50335923026608,-0.959821282999966,
0.00314634434472348));
#35716=CARTESIAN_POINT('Ctrl Pts',(-6.50312733176438,-0.959818590364428,
5.77507014088167E-5));
#35717=CARTESIAN_POINT('Origin',(-8.61687266823562,0.,0.));
#35718=CARTESIAN_POINT('',(-7.49187266823562,-0.959412934693052,0.000617836956614901));
#35719=CARTESIAN_POINT('',(-7.40312733176438,-0.956848572177365,0.000426154272836141));
#35720=CARTESIAN_POINT('',(-8.61687266823562,-0.95825,-1.32069628103871E-13));
#35721=CARTESIAN_POINT('Ctrl Pts',(-7.49187266823563,-0.959412934693052,
0.000617836956614886));
#35722=CARTESIAN_POINT('Ctrl Pts',(-7.47046414096167,-0.95745509653909,
-0.284810027720839));
#35723=CARTESIAN_POINT('Ctrl Pts',(-7.4252320861153,-0.670938943283241,
-0.891502624484874));
#35724=CARTESIAN_POINT('Ctrl Pts',(-7.35617650369652,0.360498878016349,
-1.07377985091759));
#35725=CARTESIAN_POINT('Ctrl Pts',(-7.28470592097927,1.09779410779162,-0.279175995659392));
#35726=CARTESIAN_POINT('Ctrl Pts',(-7.21323533826203,0.829645878065874,
0.771234893840035));
#35727=CARTESIAN_POINT('Ctrl Pts',(-7.14176475554478,-0.198379160483441,
1.11521820608871));
#35728=CARTESIAN_POINT('Ctrl Pts',(-7.08464386553598,-0.874781647304231,
0.573819820530738));
#35729=CARTESIAN_POINT('Ctrl Pts',(-7.05134650309959,-0.957550131185408,
0.127664759202453));
#35730=CARTESIAN_POINT('Ctrl Pts',(-7.04187266823562,-0.956941536305503,
0.000507261239360299));
#35731=CARTESIAN_POINT('Ctrl Pts',(-7.40312733176438,-0.956848572177365,
0.000426154272836167));
#35732=CARTESIAN_POINT('Ctrl Pts',(-7.38924156113507,-0.956115802214307,
-0.185995226131067));
#35733=CARTESIAN_POINT('Ctrl Pts',(-7.35153226293335,-0.813486685078433,
-0.693301032778434));
#35734=CARTESIAN_POINT('Ctrl Pts',(-7.28999943715921,0.00993354252272871,
-1.13268140760685));
#35735=CARTESIAN_POINT('Ctrl Pts',(-7.21852885444197,0.95723056012177,-0.605637750215496));
#35736=CARTESIAN_POINT('Ctrl Pts',(-7.14705827172472,1.02781206513943,0.476121036543225));
#35737=CARTESIAN_POINT('Ctrl Pts',(-7.07558768900747,0.157024683432387,
1.12179557439976));
#35738=CARTESIAN_POINT('Ctrl Pts',(-7.01094404235403,-0.760663146684144,
0.776496209154286));
#35739=CARTESIAN_POINT('Ctrl Pts',(-6.97012392327299,-0.95582027685209,
0.226801797796848));
#35740=CARTESIAN_POINT('Ctrl Pts',(-6.95312733176437,-0.957745460096,-0.000843557184232414));
#35741=CARTESIAN_POINT('Ctrl Pts',(-7.93323468161444,-0.418777734804018,
0.861898063191011));
#35742=CARTESIAN_POINT('Ctrl Pts',(-7.90941115404202,-0.705478813976586,
0.722596173989356));
#35743=CARTESIAN_POINT('Ctrl Pts',(-7.86176409889719,-1.12398839549112,
0.137840937796296));
#35744=CARTESIAN_POINT('Ctrl Pts',(-7.79029351617994,-0.724317328358726,
-0.871877473921692));
#35745=CARTESIAN_POINT('Ctrl Pts',(-7.7188229334627,0.339691526025321,-1.08024419838854));
#35746=CARTESIAN_POINT('Ctrl Pts',(-7.64735235074545,1.09209582283259,-0.300632258159738));
#35747=CARTESIAN_POINT('Ctrl Pts',(-7.5758817680282,0.844510306117659,0.755061250975084));
#35748=CARTESIAN_POINT('Ctrl Pts',(-7.50441118531095,-0.17668969425852,
1.11881329398577));
#35749=CARTESIAN_POINT('Ctrl Pts',(-7.43294060259371,-1.03599061787127,
0.458055163568042));
#35750=CARTESIAN_POINT('Ctrl Pts',(-7.36147001987646,-0.946471802875193,
-0.62233963427798));
#35751=CARTESIAN_POINT('Ctrl Pts',(-7.28999943715921,0.00993354252272871,
-1.13268140760685));
#35752=CARTESIAN_POINT('Ctrl Pts',(-7.21852885444197,0.95723056012177,-0.605637750215496));
#35753=CARTESIAN_POINT('Ctrl Pts',(-7.14705827172472,1.02781206513943,0.476121036543225));
#35754=CARTESIAN_POINT('Ctrl Pts',(-7.07558768900747,0.157024683432387,
1.12179557439976));
#35755=CARTESIAN_POINT('Ctrl Pts',(-7.00411710629023,-0.857579030410797,
0.740029567628956));
#35756=CARTESIAN_POINT('Ctrl Pts',(-6.93264652357297,-1.08673276902163,
-0.319526746285243));
#35757=CARTESIAN_POINT('Ctrl Pts',(-6.86117594085573,-0.32055498375887,
-1.08642949326629));
#35758=CARTESIAN_POINT('Ctrl Pts',(-6.78970535813849,0.739216698253442,
-0.858279536751942));
#35759=CARTESIAN_POINT('Ctrl Pts',(-6.71823477542123,1.12194498002037,0.155963109595212));
#35760=CARTESIAN_POINT('Ctrl Pts',(-6.64676419270399,0.477091470497689,
1.02736003461986));
#35761=CARTESIAN_POINT('Ctrl Pts',(-6.57529360998674,-0.604726820287475,
0.957805026523516));
#35762=CARTESIAN_POINT('Ctrl Pts',(-6.50382302726949,-1.1326799710869,0.0110028993876029));
#35763=CARTESIAN_POINT('Ctrl Pts',(-6.43235244455225,-0.623219277748515,
-0.94587668221305));
#35764=CARTESIAN_POINT('Ctrl Pts',(-6.360881861835,0.457043683047776,-1.03643429626688));
#35765=CARTESIAN_POINT('Ctrl Pts',(-6.28941127911776,1.11870346430575,-0.177728822944574));
#35766=CARTESIAN_POINT('Ctrl Pts',(-6.2179406964005,0.755750395960032,0.843757259442018));
#35767=CARTESIAN_POINT('Ctrl Pts',(-6.14647011368326,-0.299389288185346,
1.09245184324826));
#35768=CARTESIAN_POINT('Ctrl Pts',(-6.07499953096601,-1.08032037219545,
0.340577257808081));
#35769=CARTESIAN_POINT('Ctrl Pts',(-6.00352894824877,-0.871793419144197,
-0.72322970712875));
#35770=CARTESIAN_POINT('Ctrl Pts',(-5.93205836553151,0.135203161210182,
-1.12463553224998));
#35771=CARTESIAN_POINT('Ctrl Pts',(-5.86058778281427,1.01836809138401,-0.495995368476964));
#35772=CARTESIAN_POINT('Ctrl Pts',(-5.78911720009702,0.968816654749839,
0.586923559386877));
#35773=CARTESIAN_POINT('Ctrl Pts',(-5.71764661737977,0.0319326731109062,
1.13228321523766));
#35774=CARTESIAN_POINT('Ctrl Pts',(-5.64617603466253,-0.934198225340768,
0.640592421805296));
#35775=CARTESIAN_POINT('Ctrl Pts',(-5.57470545194528,-1.04470336139031,
-0.437812587534104));
#35776=CARTESIAN_POINT('Ctrl Pts',(-5.50323486922804,-0.198371837060489,
-1.11522804366184));
#35777=CARTESIAN_POINT('Ctrl Pts',(-5.43176428651079,0.829647095487569,
-0.771213765472918));
#35778=CARTESIAN_POINT('Ctrl Pts',(-5.36029370379354,1.09779793008511,0.279149923530103));
#35779=CARTESIAN_POINT('Ctrl Pts',(-5.28882312107629,0.360483152130068,
1.07384210763829));
#35780=CARTESIAN_POINT('Ctrl Pts',(-5.21735253835905,-0.706995678278174,
0.885009653055967));
#35781=CARTESIAN_POINT('Ctrl Pts',(-5.1458819556418,-1.12694200452402,-0.114397087138167));
#35782=CARTESIAN_POINT('Ctrl Pts',(-5.07441137292454,-0.514729859854887,
-1.00902831797734));
#35783=CARTESIAN_POINT('Ctrl Pts',(-5.00294079020731,0.56891984144925,-0.979497416592661));
#35784=CARTESIAN_POINT('Ctrl Pts',(-4.93147020749005,1.13149975276759,-0.0528515334991769));
#35785=CARTESIAN_POINT('Ctrl Pts',(-4.85999962477281,0.657746782740738,
0.92220070749299));
#35786=CARTESIAN_POINT('Ctrl Pts',(-4.78852904205556,-0.418431965008117,
1.05261563059162));
#35787=CARTESIAN_POINT('Ctrl Pts',(-4.71705845933831,-1.11137173909997,
0.218947100086459));
#35788=CARTESIAN_POINT('Ctrl Pts',(-4.64558787662107,-0.786413741840137,
-0.815253581256376));
#35789=CARTESIAN_POINT('Ctrl Pts',(-4.57411729390382,0.258815220585386,
-1.10276908584694));
#35790=CARTESIAN_POINT('Ctrl Pts',(-4.50264671118657,1.06699709340334,-0.380265930337164));
#35791=CARTESIAN_POINT('Ctrl Pts',(-4.43117612846933,0.897923629232473,
0.690520188823135));
#35792=CARTESIAN_POINT('Ctrl Pts',(-4.35970554575208,-0.093551942967458,
1.12886359188051));
#35793=CARTESIAN_POINT('Ctrl Pts',(-4.28823496303483,-0.999343930726676,
0.533288555311391));
#35794=CARTESIAN_POINT('Ctrl Pts',(-4.21676438031758,-0.989843650280205,
-0.550721820074632));
#35795=CARTESIAN_POINT('Ctrl Pts',(-4.14529379760033,-0.0737523434839011,
-1.1303298487331));
#35796=CARTESIAN_POINT('Ctrl Pts',(-4.07382321488309,0.909888230063614,
-0.674676503146548));
#35797=CARTESIAN_POINT('Ctrl Pts',(-4.00235263216584,1.06016839954784,0.398908435241142));
#35798=CARTESIAN_POINT('Ctrl Pts',(-3.93088204944859,0.239447586020594,
1.1071358672969));
#35799=CARTESIAN_POINT('Ctrl Pts',(-3.85941146673135,-0.80058163313813,
0.801345134001721));
#35800=CARTESIAN_POINT('Ctrl Pts',(-3.7879408840141,-1.10736361243421,-0.238392124372853));
#35801=CARTESIAN_POINT('Ctrl Pts',(-3.71647030129686,-0.399918836166434,
-1.05978766721718));
#35802=CARTESIAN_POINT('Ctrl Pts',(-3.6449997185796,0.673808865727154,-0.910530937186564));
#35803=CARTESIAN_POINT('Ctrl Pts',(-3.57352913586236,1.13039963799526,0.072674847963582));
#35804=CARTESIAN_POINT('Ctrl Pts',(-3.50205855314511,0.551665116510674,
0.989318237136875));
#35805=CARTESIAN_POINT('Ctrl Pts',(-3.43058797042786,-0.532335710452797,
0.999851822263215));
#35806=CARTESIAN_POINT('Ctrl Pts',(-3.35911738771062,-1.12877390268557,
0.0946279648007577));
#35807=CARTESIAN_POINT('Ctrl Pts',(-3.28764680499337,-0.691375801011796,
-0.897264998136924));
#35808=CARTESIAN_POINT('Ctrl Pts',(-3.21617622227613,0.379248666114025,
-1.0673590887593));
#35809=CARTESIAN_POINT('Ctrl Pts',(-3.14470563955887,1.10252187493073,-0.259866293323276));
#35810=CARTESIAN_POINT('Ctrl Pts',(-3.07323505684163,0.816002842433735,
0.785636262049064));
#35811=CARTESIAN_POINT('Ctrl Pts',(-3.00176447412438,-0.217887610001112,
1.11157994067649));
#35812=CARTESIAN_POINT('Ctrl Pts',(-2.93029389140713,-1.05221629131795,
0.419435157552917));
#35813=CARTESIAN_POINT('Ctrl Pts',(-2.85882330868989,-0.922827271139325,
-0.656867416415175));
#35814=CARTESIAN_POINT('Ctrl Pts',(-2.78735272597264,0.051772932289347,
-1.13154961826182));
#35815=CARTESIAN_POINT('Ctrl Pts',(-2.71588214325539,0.978954661287059,
-0.569853267298351));
#35816=CARTESIAN_POINT('Ctrl Pts',(-2.64441156053815,1.00951851444678,0.513767791999302));
#35817=CARTESIAN_POINT('Ctrl Pts',(-2.5729409778209,0.115471267790065,1.12683244602779));
#35818=CARTESIAN_POINT('Ctrl Pts',(-2.50147039510365,-0.884335322929965,
0.707838973018747));
#35819=CARTESIAN_POINT('Ctrl Pts',(-2.4299998123864,-1.07418524238789,-0.359459372036147));
#35820=CARTESIAN_POINT('Ctrl Pts',(-2.35852922966916,-0.280196248383438,
-1.09753133781927));
#35821=CARTESIAN_POINT('Ctrl Pts',(-2.28705864695191,0.770422572284684,
-0.830381861084687));
#35822=CARTESIAN_POINT('Ctrl Pts',(-2.21558806423466,1.11541663057547,0.197308680388403));
#35823=CARTESIAN_POINT('Ctrl Pts',(-2.14411748151742,0.438808229068046,
1.04428555155484));
#35824=CARTESIAN_POINT('Ctrl Pts',(-2.07264689880016,-0.639701626885685,
0.93480843152997));
#35825=CARTESIAN_POINT('Ctrl Pts',(-2.00117631608292,-1.13231313996798,
-0.030853334605713));
#35826=CARTESIAN_POINT('Ctrl Pts',(-1.92970573336567,-0.587846795790038,
-0.968256742613268));
#35827=CARTESIAN_POINT('Ctrl Pts',(-1.85823515064843,0.4950244060751,-1.01884042543795));
#35828=CARTESIAN_POINT('Ctrl Pts',(-1.78676456793118,1.12450614210672,-0.13627513368518));
#35829=CARTESIAN_POINT('Ctrl Pts',(-1.71529398521393,0.724060395961153,
0.871103620044959));
#35830=CARTESIAN_POINT('Ctrl Pts',(-1.64382340249668,-0.339547310642638,
1.08064452961661));
#35831=CARTESIAN_POINT('Ctrl Pts',(-1.57235281977943,-1.09216596230081,
0.300430506912404));
#35832=CARTESIAN_POINT('Ctrl Pts',(-1.50088223706219,-0.844477275441778,
-0.754945757901968));
#35833=CARTESIAN_POINT('Ctrl Pts',(-1.42941165434494,0.176662356954578,
-1.11887237535459));
#35834=CARTESIAN_POINT('Ctrl Pts',(-1.3579410716277,1.03599816963305,-0.458031427443242));
#35835=CARTESIAN_POINT('Ctrl Pts',(-1.28647048891045,0.946470301531875,
0.622317346917095));
#35836=CARTESIAN_POINT('Ctrl Pts',(-1.2149999061932,-0.00992315233657026,
1.13268996675844));
#35837=CARTESIAN_POINT('Ctrl Pts',(-1.14352932347595,-0.957228224473628,
0.60563951031527));
#35838=CARTESIAN_POINT('Ctrl Pts',(-1.07205874075871,-1.02781420127466,
-0.476111866171842));
#35839=CARTESIAN_POINT('Ctrl Pts',(-1.00058815804146,-0.157032780474456,
-1.12179595235208));
#35840=CARTESIAN_POINT('Ctrl Pts',(-0.929117575324211,0.857575021859809,
-0.740034212889895));
#35841=CARTESIAN_POINT('Ctrl Pts',(-0.857646992606967,1.0867335802145,0.31951868111913));
#35842=CARTESIAN_POINT('Ctrl Pts',(-0.786176409889718,0.320564368022132,
1.08642872230062));
#35843=CARTESIAN_POINT('Ctrl Pts',(-0.714705827172471,-0.739215298950436,
0.858282104855236));
#35844=CARTESIAN_POINT('Ctrl Pts',(-0.643235244455224,-1.12193803373525,
-0.15595157858626));
#35845=CARTESIAN_POINT('Ctrl Pts',(-0.571764661737977,-0.477113298122812,
-1.02736478175254));
#35846=CARTESIAN_POINT('Ctrl Pts',(-0.50029407902073,0.604749195542173,
-0.957794082086403));
#35847=CARTESIAN_POINT('Ctrl Pts',(-0.428823496303482,1.1326255269949,-0.0110385894026361));
#35848=CARTESIAN_POINT('Ctrl Pts',(-0.357352913586236,0.623328692801092,
0.945926260653483));
#35849=CARTESIAN_POINT('Ctrl Pts',(-0.285882330868988,-0.457232996199784,
1.03633538397604));
#35850=CARTESIAN_POINT('Ctrl Pts',(-0.214411748151741,-1.11832855125311,
0.177930077439508));
#35851=CARTESIAN_POINT('Ctrl Pts',(-0.142941165434494,-0.756478312243647,
-0.844124685575415));
#35852=CARTESIAN_POINT('Ctrl Pts',(-0.0714705827172459,0.300862454100803,
-1.09171050239691));
#35853=CARTESIAN_POINT('Ctrl Pts',(-0.0238235275724158,0.818068118928352,
-0.592123416550042));
#35854=CARTESIAN_POINT('Ctrl Pts',(0.,0.913908649078056,-0.288121577880454));
#35855=CARTESIAN_POINT('Ctrl Pts',(-7.88382312107629,-0.456179659636056,
0.93887600135061));
#35856=CARTESIAN_POINT('Ctrl Pts',(-7.85999959350388,-0.768486618303383,
0.78713276592667));
#35857=CARTESIAN_POINT('Ctrl Pts',(-7.81235253835904,-1.22437417531279,
0.150151803359993));
#35858=CARTESIAN_POINT('Ctrl Pts',(-7.74088195564181,-0.789007640231457,
-0.949746694351075));
#35859=CARTESIAN_POINT('Ctrl Pts',(-7.66941137292455,0.370030094355424,
-1.17672309148751));
#35860=CARTESIAN_POINT('Ctrl Pts',(-7.5979407902073,1.18963320956613,-0.327482360701716));
#35861=CARTESIAN_POINT('Ctrl Pts',(-7.52647020749006,0.919935306933638,
0.822497367572291));
#35862=CARTESIAN_POINT('Ctrl Pts',(-7.4549996247728,-0.192470224391866,
1.21873687455134));
#35863=CARTESIAN_POINT('Ctrl Pts',(-7.38352904205557,-1.12851713013788,
0.498965038599307));
#35864=CARTESIAN_POINT('Ctrl Pts',(-7.3120584593383,-1.03100320052307,-0.677922102701611));
#35865=CARTESIAN_POINT('Ctrl Pts',(-7.24058787662108,0.0108207282058917,
-1.23384357871844));
#35866=CARTESIAN_POINT('Ctrl Pts',(-7.16911729390382,1.04272284512438,-0.659728538064129));
#35867=CARTESIAN_POINT('Ctrl Pts',(-7.09764671118657,1.11960813357132,0.518644412882883));
#35868=CARTESIAN_POINT('Ctrl Pts',(-7.02617612846932,0.171048889875141,
1.22198550873392));
#35869=CARTESIAN_POINT('Ctrl Pts',(-6.95470554575208,-0.934171226621928,
0.806123172808106));
#35870=CARTESIAN_POINT('Ctrl Pts',(-6.88323496303483,-1.18379117008131,
-0.348064355506461));
#35871=CARTESIAN_POINT('Ctrl Pts',(-6.81176438031758,-0.349184427042679,
-1.1834608081271));
#35872=CARTESIAN_POINT('Ctrl Pts',(-6.74029379760034,0.805237704350161,
-0.934934296665356));
#35873=CARTESIAN_POINT('Ctrl Pts',(-6.66882321488309,1.22214825808638,0.169892504634269));
#35874=CARTESIAN_POINT('Ctrl Pts',(-6.59735263216585,0.519701518345439,
1.1191157312504));
#35875=CARTESIAN_POINT('Ctrl Pts',(-6.52588204944859,-0.658736251058421,
1.04334861833495));
#35876=CARTESIAN_POINT('Ctrl Pts',(-6.45441146673136,-1.23384201389987,
0.0119855915931193));
#35877=CARTESIAN_POINT('Ctrl Pts',(-6.38294088401409,-0.678880308990175,
-1.03035492837643));
#35878=CARTESIAN_POINT('Ctrl Pts',(-6.31147030129687,0.497863220615383,
-1.12900043438899));
#35879=CARTESIAN_POINT('Ctrl Pts',(-6.2399997185796,1.21861723575039,-0.193602159857718));
#35880=CARTESIAN_POINT('Ctrl Pts',(-6.16852913586237,0.823248061552785,
0.919115004067365));
#35881=CARTESIAN_POINT('Ctrl Pts',(-6.09705855314511,-0.326128378451125,
1.1900210269178));
#35882=CARTESIAN_POINT('Ctrl Pts',(-6.02558797042787,-1.17680606853814,
0.370994932716252));
#35883=CARTESIAN_POINT('Ctrl Pts',(-5.95411738771062,-0.949655132463719,
-0.787822881250074));
#35884=CARTESIAN_POINT('Ctrl Pts',(-5.88264680499338,0.147278441370431,
-1.2250791092237));
#35885=CARTESIAN_POINT('Ctrl Pts',(-5.81117622227612,1.10932069855432,-0.540293763417913));
#35886=CARTESIAN_POINT('Ctrl Pts',(-5.73970563955888,1.05534371835782,0.639342943288971));
#35887=CARTESIAN_POINT('Ctrl Pts',(-5.66823505684163,0.0347846476552195,
1.23340982294695));
#35888=CARTESIAN_POINT('Ctrl Pts',(-5.59676447412438,-1.0176334438315,0.697805085271177));
#35889=CARTESIAN_POINT('Ctrl Pts',(-5.52529389140713,-1.1380080272002,-0.476914555304986));
#35890=CARTESIAN_POINT('Ctrl Pts',(-5.45382330868989,-0.216088845205655,
-1.2148314179414));
#35891=CARTESIAN_POINT('Ctrl Pts',(-5.38235272597264,0.903744631539887,
-0.840092497287928));
#35892=CARTESIAN_POINT('Ctrl Pts',(-5.3108821432554,1.19584458407219,0.304081393350546));
#35893=CARTESIAN_POINT('Ctrl Pts',(-5.23941156053815,0.392678664543124,
1.16974921647771));
#35894=CARTESIAN_POINT('Ctrl Pts',(-5.1679409778209,-0.770138956962542,
0.964051736166549));
#35895=CARTESIAN_POINT('Ctrl Pts',(-5.09647039510366,-1.22759157741264,
-0.124614132836987));
#35896=CARTESIAN_POINT('Ctrl Pts',(-5.0249998123864,-0.560701471827329,
-1.0991467702395));
#35897=CARTESIAN_POINT('Ctrl Pts',(-4.95352922966916,0.619731275240731,
-1.06697840162099));
#35898=CARTESIAN_POINT('Ctrl Pts',(-4.88205864695191,1.23255638778736,-0.0575718156892628));
#35899=CARTESIAN_POINT('Ctrl Pts',(-4.81058806423466,0.716491538447744,
1.00456440230082));
#35900=CARTESIAN_POINT('Ctrl Pts',(-4.73911748151742,-0.455803008408689,
1.14662695789119));
#35901=CARTESIAN_POINT('Ctrl Pts',(-4.66764689880017,-1.21063069866651,
0.238501728470574));
#35902=CARTESIAN_POINT('Ctrl Pts',(-4.59617631608292,-0.856650015678725,
-0.888065602123423));
#35903=CARTESIAN_POINT('Ctrl Pts',(-4.52470573336567,0.281930555096303,
-1.20125972426461));
#35904=CARTESIAN_POINT('Ctrl Pts',(-4.45323515064843,1.16229285955041,-0.414228284494605));
#35905=CARTESIAN_POINT('Ctrl Pts',(-4.38176456793118,0.978119086856775,
0.752192006713493));
#35906=CARTESIAN_POINT('Ctrl Pts',(-4.31029398521393,-0.101907264771738,
1.22968478579835));
#35907=CARTESIAN_POINT('Ctrl Pts',(-4.23882340249669,-1.08859744988975,
0.580917683609934));
#35908=CARTESIAN_POINT('Ctrl Pts',(-4.16735281977944,-1.07824867931211,
-0.599907950104766));
#35909=CARTESIAN_POINT('Ctrl Pts',(-4.09588223706219,-0.080339321200062,
-1.23128199715025));
#35910=CARTESIAN_POINT('Ctrl Pts',(-4.02441165434494,0.991152271482454,
-0.734933287974066));
#35911=CARTESIAN_POINT('Ctrl Pts',(-3.95294107162769,1.15485428061016,0.434535790923593));
#35912=CARTESIAN_POINT('Ctrl Pts',(-3.88147048891045,0.2608331561435,1.20601651219767));
#35913=CARTESIAN_POINT('Ctrl Pts',(-3.8099999061932,-0.872083271300817,
0.872914962040671));
#35914=CARTESIAN_POINT('Ctrl Pts',(-3.73852932347595,-1.20626459773467,
-0.259683428984625));
#35915=CARTESIAN_POINT('Ctrl Pts',(-3.66705874075871,-0.435636432891633,
-1.15443954427014));
#35916=CARTESIAN_POINT('Ctrl Pts',(-3.59558815804146,0.733988160022454,
-0.991852380137317));
#35917=CARTESIAN_POINT('Ctrl Pts',(-3.52411757532421,1.23135801943897,0.0791655922768651));
#35918=CARTESIAN_POINT('Ctrl Pts',(-3.45264699260697,0.600935494339756,
1.07767634041016));
#35919=CARTESIAN_POINT('Ctrl Pts',(-3.38117640988972,-0.579879738162589,
1.08915070229317));
#35920=CARTESIAN_POINT('Ctrl Pts',(-3.30970582717247,-1.2295870862718,0.103079388389812));
#35921=CARTESIAN_POINT('Ctrl Pts',(-3.23823524445523,-0.753124035435595,
-0.977401632025656));
#35922=CARTESIAN_POINT('Ctrl Pts',(-3.16676466173798,0.413120166253078,
-1.16268718547691));
#35923=CARTESIAN_POINT('Ctrl Pts',(-3.09529407902073,1.20099043441884,-0.283075501362512));
#35924=CARTESIAN_POINT('Ctrl Pts',(-3.02382349630348,0.888881781400566,
0.855803097523826));
#35925=CARTESIAN_POINT('Ctrl Pts',(-2.95235291358623,-0.237347613085816,
1.21085749516599));
#35926=CARTESIAN_POINT('Ctrl Pts',(-2.88088233086899,-1.14619195278272,
0.456895798200539));
#35927=CARTESIAN_POINT('Ctrl Pts',(-2.80941174815174,-1.00524692567104,
-0.715533634056558));
#35928=CARTESIAN_POINT('Ctrl Pts',(-2.73794116543449,0.056396882325089,
-1.2326107068743));
#35929=CARTESIAN_POINT('Ctrl Pts',(-2.66647058271725,1.06638717169159,-0.620748067325792));
#35930=CARTESIAN_POINT('Ctrl Pts',(-2.595,1.09968074719197,0.559653479657632));
#35931=CARTESIAN_POINT('Ctrl Pts',(-2.52352941728275,0.125784250833858,
1.22747223401548));
#35932=CARTESIAN_POINT('Ctrl Pts',(-2.45205883456551,-0.963317180191378,
0.771057568139225));
#35933=CARTESIAN_POINT('Ctrl Pts',(-2.38058825184826,-1.17012299731723,
-0.391563448484618));
#35934=CARTESIAN_POINT('Ctrl Pts',(-2.30911766913101,-0.30522116768859,
-1.19555418188749));
#35935=CARTESIAN_POINT('Ctrl Pts',(-2.23764708641376,0.839230640963375,
-0.904545020605871));
#35936=CARTESIAN_POINT('Ctrl Pts',(-2.16617650369652,1.21503684795098,0.214930735763543));
#35937=CARTESIAN_POINT('Ctrl Pts',(-2.09470592097927,0.477999119689234,
1.13755290188502));
#35938=CARTESIAN_POINT('Ctrl Pts',(-2.02323533826202,-0.696834731574045,
1.01829814882551));
#35939=CARTESIAN_POINT('Ctrl Pts',(-1.95176475554478,-1.23344242031819,
-0.0336089111462738));
#35940=CARTESIAN_POINT('Ctrl Pts',(-1.88029417282753,-0.640348635887132,
-1.05473379928461));
#35941=CARTESIAN_POINT('Ctrl Pts',(-1.80882359011028,0.539236082311204,
-1.10983521776118));
#35942=CARTESIAN_POINT('Ctrl Pts',(-1.73735300739303,1.22493816297319,-0.148446153973453));
#35943=CARTESIAN_POINT('Ctrl Pts',(-1.66588242467579,0.788727760658277,
0.94890372594861));
#35944=CARTESIAN_POINT('Ctrl Pts',(-1.59441184195854,-0.369872998792028,
1.1771591771439));
#35945=CARTESIAN_POINT('Ctrl Pts',(-1.52294125924129,-1.18970961333854,
0.327262590623961));
#35946=CARTESIAN_POINT('Ctrl Pts',(-1.45147067652405,-0.919899326218264,
-0.822371559568652));
#35947=CARTESIAN_POINT('Ctrl Pts',(-1.3800000938068,0.192440445535514,-1.2188012326021));
#35948=CARTESIAN_POINT('Ctrl Pts',(-1.30852951108955,1.12852535636346,-0.498939182551021));
#35949=CARTESIAN_POINT('Ctrl Pts',(-1.2370589283723,1.0310015650916,0.677897824809409));
#35950=CARTESIAN_POINT('Ctrl Pts',(-1.16558834565506,-0.0108094100502411,
1.23385290230595));
#35951=CARTESIAN_POINT('Ctrl Pts',(-1.09411776293781,-1.04272030087456,
0.659730455362137));
#35952=CARTESIAN_POINT('Ctrl Pts',(-1.02264718022056,-1.1196104604893,-0.518634423486247));
#35953=CARTESIAN_POINT('Ctrl Pts',(-0.951176597503313,-0.171057710081155,
-1.22198592044197));
#35954=CARTESIAN_POINT('Ctrl Pts',(-0.879706014786068,0.934166860058776,
-0.806128232947122));
#35955=CARTESIAN_POINT('Ctrl Pts',(-0.808235432068819,1.18379205372353,
0.348055570023312));
#35956=CARTESIAN_POINT('Ctrl Pts',(-0.736764849351574,0.349194649434331,
1.18345996830485));
#35957=CARTESIAN_POINT('Ctrl Pts',(-0.665294266634325,-0.805236180072444,
0.934937094131386));
#35958=CARTESIAN_POINT('Ctrl Pts',(-0.593823683917079,-1.22214069141385,
-0.169879943766531));
#35959=CARTESIAN_POINT('Ctrl Pts',(-0.522353101199832,-0.519725295441906,
-1.11912090235953));
#35960=CARTESIAN_POINT('Ctrl Pts',(-0.450882518482584,0.658760624694418,
-1.04333669642703));
#35961=CARTESIAN_POINT('Ctrl Pts',(-0.379411935765336,1.2337827072909,-0.0120244691588468));
#35962=CARTESIAN_POINT('Ctrl Pts',(-0.307941353048091,0.678999496132413,
1.03040893477219));
#35963=CARTESIAN_POINT('Ctrl Pts',(-0.236470770330842,-0.498069441725224,
1.12889268803235));
#35964=CARTESIAN_POINT('Ctrl Pts',(-0.165000187613595,-1.21820883842042,
0.193821388817066));
#35965=CARTESIAN_POINT('Ctrl Pts',(-0.0935296048963485,-0.824040989578577,
-0.919515245805508));
#35966=CARTESIAN_POINT('Ctrl Pts',(-0.0220590221791003,0.327733115928909,
-1.18921347534774));
#35967=CARTESIAN_POINT('Ctrl Pts',(0.0255880329657297,0.891131512105092,
-0.645007210688402));
#35968=CARTESIAN_POINT('Ctrl Pts',(0.0494115605381455,0.995531762618636,
-0.313854325117897));
#35969=CARTESIAN_POINT('Ctrl Pts',(-7.83441156053815,-0.493581584468094,
1.01585393951021));
#35970=CARTESIAN_POINT('Ctrl Pts',(-7.81058803296573,-0.831494422630182,
0.851669357863982));
#35971=CARTESIAN_POINT('Ctrl Pts',(-7.76294097782089,-1.32475995513446,
0.162462668923692));
#35972=CARTESIAN_POINT('Ctrl Pts',(-7.69147039510366,-0.85369795210419,
-1.02761591478046));
#35973=CARTESIAN_POINT('Ctrl Pts',(-7.61999981238639,0.400368662685528,
-1.27320198458648));
#35974=CARTESIAN_POINT('Ctrl Pts',(-7.54852922966917,1.28717059629967,-0.354332463243694));
#35975=CARTESIAN_POINT('Ctrl Pts',(-7.47705864695191,0.995360307749618,
0.889933484169499));
#35976=CARTESIAN_POINT('Ctrl Pts',(-7.40558806423466,-0.208250754525212,
1.3186604551169));
#35977=CARTESIAN_POINT('Ctrl Pts',(-7.33411748151742,-1.22104364240448,
0.539874913630573));
#35978=CARTESIAN_POINT('Ctrl Pts',(-7.26264689880017,-1.11553459817094,
-0.733504571125245));
#35979=CARTESIAN_POINT('Ctrl Pts',(-7.19117631608293,0.011707913889056,
-1.33500574983004));
#35980=CARTESIAN_POINT('Ctrl Pts',(-7.11970573336567,1.12821513012698,-0.713819325912764));
#35981=CARTESIAN_POINT('Ctrl Pts',(-7.04823515064843,1.2114042020032,0.561167789222543));
#35982=CARTESIAN_POINT('Ctrl Pts',(-6.97676456793118,0.185073096317893,
1.32217544306809));
#35983=CARTESIAN_POINT('Ctrl Pts',(-6.90529398521393,-1.01076342283306,
0.872216777987256));
#35984=CARTESIAN_POINT('Ctrl Pts',(-6.83382340249668,-1.28084957114099,
-0.376601964727679));
#35985=CARTESIAN_POINT('Ctrl Pts',(-6.76235281977945,-0.377813870326487,
-1.28049212298791));
#35986=CARTESIAN_POINT('Ctrl Pts',(-6.69088223706219,0.871258710446879,
-1.01158905657877));
#35987=CARTESIAN_POINT('Ctrl Pts',(-6.61941165434495,1.32235153615238,0.183821899673327));
#35988=CARTESIAN_POINT('Ctrl Pts',(-6.54794107162769,0.562311566193189,
1.21087142788093));
#35989=CARTESIAN_POINT('Ctrl Pts',(-6.47647048891046,-0.712745681829367,
1.12889221014639));
#35990=CARTESIAN_POINT('Ctrl Pts',(-6.40499990619319,-1.33500405671283,
0.0129682837986347));
#35991=CARTESIAN_POINT('Ctrl Pts',(-6.33352932347597,-0.734541340231837,
-1.11483317453981));
#35992=CARTESIAN_POINT('Ctrl Pts',(-6.26205874075869,0.538682758182991,
-1.2215665725111));
#35993=CARTESIAN_POINT('Ctrl Pts',(-6.19058815804147,1.31853100719504,-0.209475496770861));
#35994=CARTESIAN_POINT('Ctrl Pts',(-6.11911757532421,0.890745727145539,
0.994472748692709));
#35995=CARTESIAN_POINT('Ctrl Pts',(-6.04764699260697,-0.352867468716904,
1.28759021058733));
#35996=CARTESIAN_POINT('Ctrl Pts',(-5.97617640988972,-1.27329176488084,
0.401412607624421));
#35997=CARTESIAN_POINT('Ctrl Pts',(-5.90470582717247,-1.02751684578324,
-0.852416055371398));
#35998=CARTESIAN_POINT('Ctrl Pts',(-5.83323524445523,0.159353721530679,
-1.32552268619742));
#35999=CARTESIAN_POINT('Ctrl Pts',(-5.76176466173798,1.20027330572462,-0.584592158358864));
#36000=CARTESIAN_POINT('Ctrl Pts',(-5.69029407902073,1.1418707819658,0.691762327191066));
#36001=CARTESIAN_POINT('Ctrl Pts',(-5.61882349630349,0.0376366221995333,
1.33453643065623));
#36002=CARTESIAN_POINT('Ctrl Pts',(-5.54735291358624,-1.10106866232222,
0.755017748737059));
#36003=CARTESIAN_POINT('Ctrl Pts',(-5.47588233086899,-1.23131269301009,
-0.51601652307587));
#36004=CARTESIAN_POINT('Ctrl Pts',(-5.40441174815174,-0.233805853350823,
-1.31443479222096));
#36005=CARTESIAN_POINT('Ctrl Pts',(-5.33294116543449,0.977842167592207,
-0.908971229102938));
#36006=CARTESIAN_POINT('Ctrl Pts',(-5.26147058271725,1.29389123805927,0.329012863170987));
#36007=CARTESIAN_POINT('Ctrl Pts',(-5.19,0.42487417695618,1.26565632531713));
#36008=CARTESIAN_POINT('Ctrl Pts',(-5.11852941728275,-0.833282235646911,
1.04309381927713));
#36009=CARTESIAN_POINT('Ctrl Pts',(-5.04705883456551,-1.32824115030125,
-0.134831178535808));
#36010=CARTESIAN_POINT('Ctrl Pts',(-4.97558825184826,-0.606673083799771,
-1.18926522250167));
#36011=CARTESIAN_POINT('Ctrl Pts',(-4.90411766913101,0.670542709032212,
-1.15445938664932));
#36012=CARTESIAN_POINT('Ctrl Pts',(-4.83264708641377,1.33361302280713,-0.0622920978793508));
#36013=CARTESIAN_POINT('Ctrl Pts',(-4.76117650369652,0.77523629415475,1.08692809710864));
#36014=CARTESIAN_POINT('Ctrl Pts',(-4.68970592097927,-0.493174051809261,
1.24063828519075));
#36015=CARTESIAN_POINT('Ctrl Pts',(-4.61823533826202,-1.30988965823305,
0.25805635685469));
#36016=CARTESIAN_POINT('Ctrl Pts',(-4.54676475554478,-0.926886289517314,
-0.960877622990471));
#36017=CARTESIAN_POINT('Ctrl Pts',(-4.47529417282753,0.30504588960722,-1.29975036268229));
#36018=CARTESIAN_POINT('Ctrl Pts',(-4.40382359011029,1.25758862569748,-0.448190638652046));
#36019=CARTESIAN_POINT('Ctrl Pts',(-4.33235300739303,1.05831454448108,0.81386382460385));
#36020=CARTESIAN_POINT('Ctrl Pts',(-4.26088242467579,-0.110262586576019,
1.3305059797162));
#36021=CARTESIAN_POINT('Ctrl Pts',(-4.18941184195854,-1.17785096905283,
0.628546811908475));
#36022=CARTESIAN_POINT('Ctrl Pts',(-4.11794125924129,-1.16665370834401,
-0.649094080134899));
#36023=CARTESIAN_POINT('Ctrl Pts',(-4.04647067652405,-0.0869262989162214,
-1.33223414556741));
#36024=CARTESIAN_POINT('Ctrl Pts',(-3.9750000938068,1.07241631290129,-0.795190072801583));
#36025=CARTESIAN_POINT('Ctrl Pts',(-3.90352951108955,1.24954016167249,0.470163146606043));
#36026=CARTESIAN_POINT('Ctrl Pts',(-3.83205892837231,0.282218726266407,
1.30489715709843));
#36027=CARTESIAN_POINT('Ctrl Pts',(-3.76058834565505,-0.943584909463504,
0.94448479007962));
#36028=CARTESIAN_POINT('Ctrl Pts',(-3.68911776293781,-1.30516558303513,
-0.280974733596397));
#36029=CARTESIAN_POINT('Ctrl Pts',(-3.61764718022056,-0.471354029616834,
-1.24909142132311));
#36030=CARTESIAN_POINT('Ctrl Pts',(-3.54617659750332,0.794167454317755,
-1.07317382308807));
#36031=CARTESIAN_POINT('Ctrl Pts',(-3.47470601478607,1.33231640088267,0.0856563365901476));
#36032=CARTESIAN_POINT('Ctrl Pts',(-3.40323543206882,0.650205872168837,
1.16603444368344));
#36033=CARTESIAN_POINT('Ctrl Pts',(-3.33176484935158,-0.627423765872378,
1.17844958232312));
#36034=CARTESIAN_POINT('Ctrl Pts',(-3.26029426663432,-1.33040026985804,
0.111530811978866));
#36035=CARTESIAN_POINT('Ctrl Pts',(-3.18882368391708,-0.814872269859391,
-1.05753826591439));
#36036=CARTESIAN_POINT('Ctrl Pts',(-3.11735310119983,0.44699166639213,-1.25801528219453));
#36037=CARTESIAN_POINT('Ctrl Pts',(-3.04588251848259,1.29945899390695,-0.306284709401745));
#36038=CARTESIAN_POINT('Ctrl Pts',(-2.97441193576534,0.961760720367394,
0.925969932998585));
#36039=CARTESIAN_POINT('Ctrl Pts',(-2.90294135304809,-0.256807616170518,
1.3101350496555));
#36040=CARTESIAN_POINT('Ctrl Pts',(-2.83147077033084,-1.2401676142475,0.49435643884816));
#36041=CARTESIAN_POINT('Ctrl Pts',(-2.7600001876136,-1.08766658020275,-0.77419985169794));
#36042=CARTESIAN_POINT('Ctrl Pts',(-2.68852960489635,0.061020832360832,
-1.33367179548678));
#36043=CARTESIAN_POINT('Ctrl Pts',(-2.6170590221791,1.15381968209612,-0.671642867353233));
#36044=CARTESIAN_POINT('Ctrl Pts',(-2.54558843946185,1.18984297993716,0.605539167315962));
#36045=CARTESIAN_POINT('Ctrl Pts',(-2.47411785674461,0.136097233877648,
1.32811202200318));
#36046=CARTESIAN_POINT('Ctrl Pts',(-2.40264727402736,-1.04229903745279,
0.834276163259703));
#36047=CARTESIAN_POINT('Ctrl Pts',(-2.33117669131011,-1.26606075224656,
-0.423667524933089));
#36048=CARTESIAN_POINT('Ctrl Pts',(-2.25970610859287,-0.330246086993743,
-1.2935770259557));
#36049=CARTESIAN_POINT('Ctrl Pts',(-2.18823552587562,0.908038709642064,
-0.978708180127054));
#36050=CARTESIAN_POINT('Ctrl Pts',(-2.11676494315837,1.3146570653265,0.232552791138683));
#36051=CARTESIAN_POINT('Ctrl Pts',(-2.04529436044112,0.517190010310421,
1.2308202522152));
#36052=CARTESIAN_POINT('Ctrl Pts',(-1.97382377772388,-0.753967836262407,
1.10178786612104));
#36053=CARTESIAN_POINT('Ctrl Pts',(-1.90235319500663,-1.3345717006684,-0.0363644876868344));
#36054=CARTESIAN_POINT('Ctrl Pts',(-1.83088261228938,-0.692850475984229,
-1.14121085595595));
#36055=CARTESIAN_POINT('Ctrl Pts',(-1.75941202957214,0.583447758547311,
-1.20083001008441));
#36056=CARTESIAN_POINT('Ctrl Pts',(-1.68794144685489,1.32537018383966,-0.160617174261725));
#36057=CARTESIAN_POINT('Ctrl Pts',(-1.61647086413764,0.853395125355401,
1.02670383185226));
#36058=CARTESIAN_POINT('Ctrl Pts',(-1.54500028142039,-0.400198686941418,
1.27367382467119));
#36059=CARTESIAN_POINT('Ctrl Pts',(-1.47352969870315,-1.28725326437627,
0.354094674335519));
#36060=CARTESIAN_POINT('Ctrl Pts',(-1.4020591159859,-0.995321376994749,
-0.889797361235337));
#36061=CARTESIAN_POINT('Ctrl Pts',(-1.33058853326865,0.20821853411645,-1.31873008984962));
#36062=CARTESIAN_POINT('Ctrl Pts',(-1.2591179505514,1.22105254309388,-0.539846937658801));
#36063=CARTESIAN_POINT('Ctrl Pts',(-1.18764736783416,1.11553282865133,0.733478302701723));
#36064=CARTESIAN_POINT('Ctrl Pts',(-1.11617678511691,-0.0116956677639116,
1.33501583785347));
#36065=CARTESIAN_POINT('Ctrl Pts',(-1.04470620239966,-1.12821237727549,
0.713821400409003));
#36066=CARTESIAN_POINT('Ctrl Pts',(-0.973235619682415,-1.21140671970395,
-0.561156980800651));
#36067=CARTESIAN_POINT('Ctrl Pts',(-0.90176503696517,-0.185082639687852,
-1.32217588853185));
#36068=CARTESIAN_POINT('Ctrl Pts',(-0.830294454247922,1.01075869825774,
-0.872222253004347));
#36069=CARTESIAN_POINT('Ctrl Pts',(-0.758823871530675,1.28085052723256,
0.376592458927494));
#36070=CARTESIAN_POINT('Ctrl Pts',(-0.687353288813427,0.37782493084653,
1.28049121430909));
#36071=CARTESIAN_POINT('Ctrl Pts',(-0.61588270609618,-0.871257061194453,
1.01159208340753));
#36072=CARTESIAN_POINT('Ctrl Pts',(-0.544412123378933,-1.32234334909244,
-0.1838083089468));
#36073=CARTESIAN_POINT('Ctrl Pts',(-0.472941540661686,-0.562337292761001,
-1.21087702296652));
#36074=CARTESIAN_POINT('Ctrl Pts',(-0.401470957944439,0.712772053846664,
-1.12887931076765));
#36075=CARTESIAN_POINT('Ctrl Pts',(-0.330000375227191,1.33493988758691,
-0.0130103489150566));
#36076=CARTESIAN_POINT('Ctrl Pts',(-0.258529792509945,0.734670299463734,
1.1148916088909));
#36077=CARTESIAN_POINT('Ctrl Pts',(-0.187059209792697,-0.538905887250664,
1.22144999208865));
#36078=CARTESIAN_POINT('Ctrl Pts',(-0.11558862707545,-1.31808912558773,
0.209712700194622));
#36079=CARTESIAN_POINT('Ctrl Pts',(-0.044118044358203,-0.891603666913505,
-0.994905806035601));
#36080=CARTESIAN_POINT('Ctrl Pts',(0.0273525383590451,0.354603777757012,
-1.28671644829858));
#36081=CARTESIAN_POINT('Ctrl Pts',(0.0749995935038751,0.964194905281832,
-0.697891004826763));
#36082=CARTESIAN_POINT('Ctrl Pts',(0.0988231210762909,1.07715487615921,
-0.33958707235534));
#36083=CARTESIAN_POINT('Ctrl Pts',(-7.785,-0.530983509300131,1.09283187766981));
#36084=CARTESIAN_POINT('Ctrl Pts',(-7.76117647242759,-0.89450222695698,
0.916205949801296));
#36085=CARTESIAN_POINT('Ctrl Pts',(-7.71352941728276,-1.42514573495613,
0.174773534487387));
#36086=CARTESIAN_POINT('Ctrl Pts',(-7.6420588345655,-0.918388263976919,
-1.10548513520984));
#36087=CARTESIAN_POINT('Ctrl Pts',(-7.57058825184826,0.43070723101563,-1.36968087768545));
#36088=CARTESIAN_POINT('Ctrl Pts',(-7.499117669131,1.38470798303322,-0.381182565785671));
#36089=CARTESIAN_POINT('Ctrl Pts',(-7.42764708641377,1.0707853085656,0.957369600766706));
#36090=CARTESIAN_POINT('Ctrl Pts',(-7.35617650369651,-0.224031284658557,
1.41858403568246));
#36091=CARTESIAN_POINT('Ctrl Pts',(-7.28470592097928,-1.31357015467109,
0.580784788661838));
#36092=CARTESIAN_POINT('Ctrl Pts',(-7.21323533826202,-1.20006599581882,
-0.789087039548876));
#36093=CARTESIAN_POINT('Ctrl Pts',(-7.14176475554478,0.0125950995722171,
-1.43616792094163));
#36094=CARTESIAN_POINT('Ctrl Pts',(-7.07029417282752,1.21370741512959,-0.767910113761398));
#36095=CARTESIAN_POINT('Ctrl Pts',(-6.99882359011029,1.30320027043509,0.603691165562203));
#36096=CARTESIAN_POINT('Ctrl Pts',(-6.92735300739303,0.199097302760646,
1.42236537740225));
#36097=CARTESIAN_POINT('Ctrl Pts',(-6.85588242467579,-1.08735561904419,
0.938310383166409));
#36098=CARTESIAN_POINT('Ctrl Pts',(-6.78441184195853,-1.37790797220067,
-0.405139573948898));
#36099=CARTESIAN_POINT('Ctrl Pts',(-6.7129412592413,-0.406443313610296,
-1.37752343784872));
#36100=CARTESIAN_POINT('Ctrl Pts',(-6.64147067652404,0.937279716543598,
-1.08824381649219));
#36101=CARTESIAN_POINT('Ctrl Pts',(-6.5700000938068,1.42255481421838,0.197751294712385));
#36102=CARTESIAN_POINT('Ctrl Pts',(-6.49852951108955,0.604921614040939,
1.30262712451147));
#36103=CARTESIAN_POINT('Ctrl Pts',(-6.4270589283723,-0.766755112600313,
1.21443580195783));
#36104=CARTESIAN_POINT('Ctrl Pts',(-6.35558834565506,-1.43616609952579,
0.0139509760041505));
#36105=CARTESIAN_POINT('Ctrl Pts',(-6.28411776293781,-0.790202371473498,
-1.19931142070319));
#36106=CARTESIAN_POINT('Ctrl Pts',(-6.21264718022056,0.579502295750599,
-1.31413271063321));
#36107=CARTESIAN_POINT('Ctrl Pts',(-6.14117659750332,1.41844477863968,-0.225348833684005));
#36108=CARTESIAN_POINT('Ctrl Pts',(-6.06970601478607,0.958243392738293,
1.06983049331806));
#36109=CARTESIAN_POINT('Ctrl Pts',(-5.99823543206882,-0.379606558982684,
1.38515939425687));
#36110=CARTESIAN_POINT('Ctrl Pts',(-5.92676484935158,-1.36977746122354,
0.431830282532593));
#36111=CARTESIAN_POINT('Ctrl Pts',(-5.85529426663433,-1.10537855910276,
-0.917009229492723));
#36112=CARTESIAN_POINT('Ctrl Pts',(-5.78382368391709,0.171429001690927,
-1.42596626317113));
#36113=CARTESIAN_POINT('Ctrl Pts',(-5.71235310119983,1.29122591289492,-0.628890553299815));
#36114=CARTESIAN_POINT('Ctrl Pts',(-5.64088251848259,1.22839784557378,0.74418171109316));
#36115=CARTESIAN_POINT('Ctrl Pts',(-5.56941193576534,0.0404885967438472,
1.43566303836552));
#36116=CARTESIAN_POINT('Ctrl Pts',(-5.49794135304809,-1.18450388081295,
0.81223041220294));
#36117=CARTESIAN_POINT('Ctrl Pts',(-5.42647077033085,-1.32461735881998,
-0.555118490846752));
#36118=CARTESIAN_POINT('Ctrl Pts',(-5.3550001876136,-0.251522861495992,
-1.41403816650052));
#36119=CARTESIAN_POINT('Ctrl Pts',(-5.28352960489635,1.05193970364453,-0.977849960917949));
#36120=CARTESIAN_POINT('Ctrl Pts',(-5.2120590221791,1.39193789204635,0.353944332991429));
#36121=CARTESIAN_POINT('Ctrl Pts',(-5.14058843946187,0.457069689369236,
1.36156343415655));
#36122=CARTESIAN_POINT('Ctrl Pts',(-5.0691178567446,-0.896425514331279,
1.12213590238771));
#36123=CARTESIAN_POINT('Ctrl Pts',(-4.99764727402737,-1.42889072318987,
-0.145048224234627));
#36124=CARTESIAN_POINT('Ctrl Pts',(-4.92617669131011,-0.652644695772212,
-1.27938367476384));
#36125=CARTESIAN_POINT('Ctrl Pts',(-4.85470610859287,0.721354142823692,
-1.24194037167764));
#36126=CARTESIAN_POINT('Ctrl Pts',(-4.78323552587561,1.4346696578269,-0.0670123800694382));
#36127=CARTESIAN_POINT('Ctrl Pts',(-4.71176494315838,0.833981049861757,
1.16929179191647));
#36128=CARTESIAN_POINT('Ctrl Pts',(-4.64029436044112,-0.530545095209834,
1.33464961249031));
#36129=CARTESIAN_POINT('Ctrl Pts',(-4.56882377772388,-1.40914861779958,
0.277610985238807));
#36130=CARTESIAN_POINT('Ctrl Pts',(-4.49735319500663,-0.997122563355904,
-1.03368964385752));
#36131=CARTESIAN_POINT('Ctrl Pts',(-4.42588261228939,0.328161224118138,
-1.39824100109996));
#36132=CARTESIAN_POINT('Ctrl Pts',(-4.35441202957214,1.35288439184455,-0.482152992809488));
#36133=CARTESIAN_POINT('Ctrl Pts',(-4.28294144685489,1.13851000210538,0.875535642494211));
#36134=CARTESIAN_POINT('Ctrl Pts',(-4.21147086413764,-0.118617908380299,
1.43132717363404));
#36135=CARTESIAN_POINT('Ctrl Pts',(-4.14000028142039,-1.26710448821591,
0.676175940207019));
#36136=CARTESIAN_POINT('Ctrl Pts',(-4.06852969870315,-1.25505873737591,
-0.698280210165035));
#36137=CARTESIAN_POINT('Ctrl Pts',(-3.9970591159859,-0.0935132766323821,
-1.43318629398456));
#36138=CARTESIAN_POINT('Ctrl Pts',(-3.92558853326866,1.15368035432013,-0.855446857629104));
#36139=CARTESIAN_POINT('Ctrl Pts',(-3.8541179505514,1.34422604273481,0.505790502288495));
#36140=CARTESIAN_POINT('Ctrl Pts',(-3.78264736783416,0.303604296389314,
1.4037778019992));
#36141=CARTESIAN_POINT('Ctrl Pts',(-3.71117678511691,-1.01508654762619,
1.01605461811857));
#36142=CARTESIAN_POINT('Ctrl Pts',(-3.63970620239967,-1.40406656833559,
-0.302266038208169));
#36143=CARTESIAN_POINT('Ctrl Pts',(-3.56823561968241,-0.507071626342034,
-1.34374329837606));
#36144=CARTESIAN_POINT('Ctrl Pts',(-3.49676503696517,0.854346748613055,
-1.15449526603882));
#36145=CARTESIAN_POINT('Ctrl Pts',(-3.42529445424792,1.43327478232637,0.0921470809034307));
#36146=CARTESIAN_POINT('Ctrl Pts',(-3.35382387153068,0.699476249997918,
1.25439254695673));
#36147=CARTESIAN_POINT('Ctrl Pts',(-3.28235328881343,-0.67496779358217,
1.26774846235307));
#36148=CARTESIAN_POINT('Ctrl Pts',(-3.21088270609618,-1.43121345344427,
0.119982235567921));
#36149=CARTESIAN_POINT('Ctrl Pts',(-3.13941212337893,-0.87662050428319,
-1.13767489980312));
#36150=CARTESIAN_POINT('Ctrl Pts',(-3.06794154066169,0.480863166531182,
-1.35334337891214));
#36151=CARTESIAN_POINT('Ctrl Pts',(-2.99647095794444,1.39792755339507,-0.32949391744098));
#36152=CARTESIAN_POINT('Ctrl Pts',(-2.9250003752272,1.03463965933422,0.996136768473347));
#36153=CARTESIAN_POINT('Ctrl Pts',(-2.85352979250994,-0.276267619255219,
1.409412604145));
#36154=CARTESIAN_POINT('Ctrl Pts',(-2.7820592097927,-1.33414327571228,0.531817079495782));
#36155=CARTESIAN_POINT('Ctrl Pts',(-2.71058862707545,-1.17008623473447,
-0.832866069339323));
#36156=CARTESIAN_POINT('Ctrl Pts',(-2.63911804435821,0.0656447823965748,
-1.43473288409926));
#36157=CARTESIAN_POINT('Ctrl Pts',(-2.56764746164095,1.24125219250066,-0.722537667380674));
#36158=CARTESIAN_POINT('Ctrl Pts',(-2.49617687892371,1.28000521268235,0.651424854974292));
#36159=CARTESIAN_POINT('Ctrl Pts',(-2.42470629620646,0.146410216921439,
1.42875180999087));
#36160=CARTESIAN_POINT('Ctrl Pts',(-2.35323571348922,-1.1212808947142,0.897494758380182));
#36161=CARTESIAN_POINT('Ctrl Pts',(-2.28176513077196,-1.3619985071759,-0.455771601381561));
#36162=CARTESIAN_POINT('Ctrl Pts',(-2.21029454805472,-0.355271006298895,
-1.39159987002391));
#36163=CARTESIAN_POINT('Ctrl Pts',(-2.13882396533747,0.976846778320755,
-1.05287133964824));
#36164=CARTESIAN_POINT('Ctrl Pts',(-2.06735338262022,1.41427728270201,0.250174846513822));
#36165=CARTESIAN_POINT('Ctrl Pts',(-1.99588279990298,0.556380900931609,
1.32408760254539));
#36166=CARTESIAN_POINT('Ctrl Pts',(-1.92441221718573,-0.811100940950769,
1.18527758341658));
#36167=CARTESIAN_POINT('Ctrl Pts',(-1.85294163446849,-1.43570098101862,
-0.0391200642273951));
#36168=CARTESIAN_POINT('Ctrl Pts',(-1.78147105175124,-0.745352316081325,
-1.22768791262729));
#36169=CARTESIAN_POINT('Ctrl Pts',(-1.71000046903399,0.627659434783417,
-1.29182480240764));
#36170=CARTESIAN_POINT('Ctrl Pts',(-1.63852988631674,1.42580220470614,-0.172788194549996));
#36171=CARTESIAN_POINT('Ctrl Pts',(-1.5670593035995,0.918062490052525,1.10450393775591));
#36172=CARTESIAN_POINT('Ctrl Pts',(-1.49558872088225,-0.430524375090808,
1.37018847219848));
#36173=CARTESIAN_POINT('Ctrl Pts',(-1.424118138165,-1.38479691541401,0.380926758047075));
#36174=CARTESIAN_POINT('Ctrl Pts',(-1.35264755544775,-1.07074342777124,
-0.957223162902021));
#36175=CARTESIAN_POINT('Ctrl Pts',(-1.28117697273051,0.223996622697387,
-1.41865894709713));
#36176=CARTESIAN_POINT('Ctrl Pts',(-1.20970639001326,1.3135797298243,-0.58075469276658));
#36177=CARTESIAN_POINT('Ctrl Pts',(-1.13823580729601,1.20006409221106,0.789058780594037));
#36178=CARTESIAN_POINT('Ctrl Pts',(-1.06676522457877,-0.0125819254775816,
1.43617877340099));
#36179=CARTESIAN_POINT('Ctrl Pts',(-0.995294641861518,-1.21370445367643,
0.767912345455868));
#36180=CARTESIAN_POINT('Ctrl Pts',(-0.92382405914427,-1.30320297891858,
-0.603679538115054));
#36181=CARTESIAN_POINT('Ctrl Pts',(-0.852353476427024,-0.199107569294552,
-1.42236585662174));
#36182=CARTESIAN_POINT('Ctrl Pts',(-0.780882893709775,1.08735053645671,
-0.938316273061573));
#36183=CARTESIAN_POINT('Ctrl Pts',(-0.70941231099253,1.37790900074158,0.405129347831677));
#36184=CARTESIAN_POINT('Ctrl Pts',(-0.637941728275282,0.406455212258731,
1.37752246031332));
#36185=CARTESIAN_POINT('Ctrl Pts',(-0.566471145558034,-0.937277942316462,
1.08824707268368));
#36186=CARTESIAN_POINT('Ctrl Pts',(-0.495000562840789,-1.42254600677103,
-0.197736674127072));
#36187=CARTESIAN_POINT('Ctrl Pts',(-0.42352998012354,-0.604949290080097,
-1.30263314357351));
#36188=CARTESIAN_POINT('Ctrl Pts',(-0.352059397406293,0.766783482998911,
-1.21442192510827));
#36189=CARTESIAN_POINT('Ctrl Pts',(-0.280588814689045,1.43609706788291,
-0.0139962286712674));
#36190=CARTESIAN_POINT('Ctrl Pts',(-0.209118231971799,0.790341102795055,
1.19937428300961));
#36191=CARTESIAN_POINT('Ctrl Pts',(-0.137647649254551,-0.579742332776104,
1.31400729614496));
#36192=CARTESIAN_POINT('Ctrl Pts',(-0.0661770665373043,-1.41796941275505,
0.22560401157218));
#36193=CARTESIAN_POINT('Ctrl Pts',(0.00529351617994245,-0.959166344248434,
-1.0702963662657));
#36194=CARTESIAN_POINT('Ctrl Pts',(0.0767640988971906,0.381474439585117,
-1.38421942124942));
#36195=CARTESIAN_POINT('Ctrl Pts',(0.124411154042021,1.03725829845857,-0.750774798965123));
#36196=CARTESIAN_POINT('Ctrl Pts',(0.148234681614436,1.15877798969979,-0.365319819592783));
#36197=CARTESIAN_POINT('',(3.3695633096113E-15,-0.876371264439109,-0.844383392149627));
#36198=CARTESIAN_POINT('Ctrl Pts',(-1.66533453693773E-16,-0.876385019502678,
-0.844404278593171));
#36199=CARTESIAN_POINT('Ctrl Pts',(-1.66201775279586E-16,-0.853668716120764,
-0.863815852990219));
#36200=CARTESIAN_POINT('Ctrl Pts',(-4.86302334741944E-16,-0.830222915225709,
-0.882299336152847));
#36201=CARTESIAN_POINT('Ctrl Pts',(-3.33066907387547E-16,-0.806064413927853,
-0.899791837105119));
#36202=CARTESIAN_POINT('Ctrl Pts',(-8.90510441733197E-17,-0.767426558861498,
-0.927768436655273));
#36203=CARTESIAN_POINT('Ctrl Pts',(-1.71711545508733E-15,-0.726965954730414,
-0.953212246495642));
#36204=CARTESIAN_POINT('Ctrl Pts',(-1.80411241501588E-15,-0.684965814764286,
-0.976084216881709));
#36205=CARTESIAN_POINT('Ctrl Pts',(-1.85091247889602E-15,-0.662371815675076,
-0.988388206308602));
#36206=CARTESIAN_POINT('Ctrl Pts',(8.90055551083889E-16,-0.639332066021806,
-0.999947230709396));
#36207=CARTESIAN_POINT('Ctrl Pts',(1.0547118733939E-15,-0.615890017093324,
-1.01075029848142));
#36208=CARTESIAN_POINT('Ctrl Pts',(1.12586562016508E-15,-0.605759889140421,
-1.01541868131554));
#36209=CARTESIAN_POINT('Ctrl Pts',(1.07131306105525E-15,-0.595554774413637,
-1.01994564355146));
#36210=CARTESIAN_POINT('Ctrl Pts',(9.15933995315754E-16,-0.585291173178408,
-1.02432501098259));
#36211=CARTESIAN_POINT('Ctrl Pts',(2.2127133981659E-16,-0.539405065837525,
-1.04390411576504));
#36212=CARTESIAN_POINT('Ctrl Pts',(-1.96359358092282E-15,-0.49228587059037,
-1.06056774636267));
#36213=CARTESIAN_POINT('Ctrl Pts',(-2.95596880306448E-15,-0.44425982933865,
-1.07426808122273));
#36214=CARTESIAN_POINT('Ctrl Pts',(-3.57545733071877E-15,-0.414279655589566,
-1.08282049172379));
#36215=CARTESIAN_POINT('Ctrl Pts',(-9.63093987522759E-16,-0.383945872099603,
-1.09021711713024));
#36216=CARTESIAN_POINT('Ctrl Pts',(-8.74300631892311E-16,-0.353338310232677,
-1.09643602014208));
#36217=CARTESIAN_POINT('Ctrl Pts',(-8.32779690395146E-16,-0.33902581154824,
-1.09934406102304));
#36218=CARTESIAN_POINT('Ctrl Pts',(-4.61009343396251E-16,-0.324653469259868,
-1.1019944657249));
#36219=CARTESIAN_POINT('Ctrl Pts',(-3.33066907387547E-16,-0.310229613717086,
-1.10438439507686));
#36220=CARTESIAN_POINT('Ctrl Pts',(-2.47338154619976E-16,-0.300564805195711,
-1.10598578449024));
#36221=CARTESIAN_POINT('Ctrl Pts',(-1.61299260203782E-15,-0.290881931078401,
-1.10746931579312));
#36222=CARTESIAN_POINT('Ctrl Pts',(-1.63757896132211E-15,-0.281191356984365,
-1.108833510341));
#36223=CARTESIAN_POINT('Ctrl Pts',(-1.7595790972034E-15,-0.233105695233064,
-1.11560278912219));
#36224=CARTESIAN_POINT('Ctrl Pts',(-1.19024471319125E-15,-0.184770819851817,
-1.11944780780858));
#36225=CARTESIAN_POINT('Ctrl Pts',(-1.20736753927986E-15,-0.136487869923575,
-1.1203187821722));
#36226=CARTESIAN_POINT('Ctrl Pts',(-1.2240112256568E-15,-0.0895559982920508,
-1.12116538448396));
#36227=CARTESIAN_POINT('Ctrl Pts',(-2.22001881418049E-15,-0.0426721509549466,
-1.11920180597511));
#36228=CARTESIAN_POINT('Ctrl Pts',(-2.08166817117217E-15,0.0038740908008012,
-1.11433562929591));
#36229=CARTESIAN_POINT('Ctrl Pts',(-2.00950571302812E-15,0.0281521942445265,
-1.11179747505753));
#36230=CARTESIAN_POINT('Ctrl Pts',(-7.50224596214795E-16,0.0523381381697833,
-1.1084688905888));
#36231=CARTESIAN_POINT('Ctrl Pts',(-1.11022302462516E-15,0.0763879906706078,
-1.10433182603949));
#36232=CARTESIAN_POINT('Ctrl Pts',(-1.32231052695403E-15,0.0905565890469971,
-1.10189453849045));
#36233=CARTESIAN_POINT('Ctrl Pts',(1.23352088475356E-15,0.10467791009547,
-1.09917658032639));
#36234=CARTESIAN_POINT('Ctrl Pts',(1.40165656858926E-15,0.118742544221765,
-1.09617371376713));
#36235=CARTESIAN_POINT('Ctrl Pts',(1.5055427343467E-15,0.127432673995702,
-1.09431832955596));
#36236=CARTESIAN_POINT('Ctrl Pts',(-2.67693673802542E-16,0.136100883638701,
-1.09235410866341));
#36237=CARTESIAN_POINT('Ctrl Pts',(-3.33066907387547E-16,0.144731539974336,
-1.09028355436426));
#36238=CARTESIAN_POINT('Ctrl Pts',(-6.67218484523858E-16,0.188846650519144,
-1.07970003345418));
#36239=CARTESIAN_POINT('Ctrl Pts',(-3.27749510057336E-15,0.232073502898363,
-1.0663233603394));
#36240=CARTESIAN_POINT('Ctrl Pts',(-2.98372437868011E-15,0.274146266817965,
-1.05007992390509));
#36241=CARTESIAN_POINT('Ctrl Pts',(-2.95431841155954E-15,0.278357681435861,
-1.04845398257699));
#36242=CARTESIAN_POINT('Ctrl Pts',(-9.03487711860832E-16,0.282557511928685,
-1.0467992790516));
#36243=CARTESIAN_POINT('Ctrl Pts',(-8.88178419700125E-16,0.286745476895236,
-1.04511571412866));
#36244=CARTESIAN_POINT('Ctrl Pts',(-7.16151853340391E-16,0.3264740599549,
-1.02914479521899));
#36245=CARTESIAN_POINT('Ctrl Pts',(-2.16871884646574E-15,0.365137127092165,
-1.01057884773605));
#36246=CARTESIAN_POINT('Ctrl Pts',(-2.4980018054066E-15,0.402568927230115,
-0.989600059824713));
#36247=CARTESIAN_POINT('Ctrl Pts',(-2.66197985924992E-15,0.421209411263105,
-0.97915293305946));
#36248=CARTESIAN_POINT('Ctrl Pts',(-1.4513023456678E-15,0.439544124644693,
-0.968107023694203));
#36249=CARTESIAN_POINT('Ctrl Pts',(-1.49880108324396E-15,0.457549730619664,
-0.956482776639175));
#36250=CARTESIAN_POINT('Ctrl Pts',(-1.53878850873768E-15,0.472707982483494,
-0.946696754173037));
#36251=CARTESIAN_POINT('Ctrl Pts',(-4.68193304594181E-16,0.487632955649028,
-0.936500815894636));
#36252=CARTESIAN_POINT('Ctrl Pts',(-6.52256026967279E-16,0.502309521134179,
-0.925906648036467));
#36253=CARTESIAN_POINT('Ctrl Pts',(-7.40772485187387E-16,0.509367536895501,
-0.920811872709318));
#36254=CARTESIAN_POINT('Ctrl Pts',(-2.46291782561222E-15,0.516359973174507,
-0.91563084291723));
#36255=CARTESIAN_POINT('Ctrl Pts',(-2.42861286636753E-15,0.523284879313264,
-0.910365918516622));
#36256=CARTESIAN_POINT('Ctrl Pts',(-2.25061356671081E-15,0.559216373476985,
-0.883047627613864));
#36257=CARTESIAN_POINT('Ctrl Pts',(-2.96823005161294E-16,0.593340067182582,
-0.853468264465714));
#36258=CARTESIAN_POINT('Ctrl Pts',(-6.03683769639929E-16,0.625471482738123,
-0.821855359183385));
#36259=CARTESIAN_POINT('Ctrl Pts',(-9.08089369103446E-16,0.657345817765653,
-0.790495385875619));
#36260=CARTESIAN_POINT('Ctrl Pts',(2.15765114517466E-16,0.687260208276574,
-0.757133177797282));
#36261=CARTESIAN_POINT('Ctrl Pts',(5.89805981832114E-16,0.714989723653526,
-0.721967245339149));
#36262=CARTESIAN_POINT('Ctrl Pts',(7.57871803351495E-16,0.727449281390145,
-0.70616632131044));
#36263=CARTESIAN_POINT('Ctrl Pts',(1.44173626698327E-16,0.739467070861113,
-0.690001019680507));
#36264=CARTESIAN_POINT('Ctrl Pts',(1.59594559789866E-16,0.751019236986007,
-0.673488664556055));
#36265=CARTESIAN_POINT('Ctrl Pts',(1.69123973183035E-16,0.758157933842884,
-0.663284803535346));
#36266=CARTESIAN_POINT('Ctrl Pts',(-8.8777281847663E-16,0.765118780990856,
-0.652948409395475));
#36267=CARTESIAN_POINT('Ctrl Pts',(-9.47159017883337E-16,0.771895701092293,
-0.642483556554596));
#36268=CARTESIAN_POINT('Ctrl Pts',(-9.8353236423952E-16,0.77604648468411,
-0.636073957678923));
#36269=CARTESIAN_POINT('Ctrl Pts',(-6.35014032128769E-16,0.780127059785162,
-0.629617905044286));
#36270=CARTESIAN_POINT('Ctrl Pts',(-6.90419943438769E-16,0.784131582650059,
-0.623124085326683));
#36271=CARTESIAN_POINT('Ctrl Pts',(-1.0034507112653E-15,0.806756223911961,
-0.586435484340496));
#36272=CARTESIAN_POINT('Ctrl Pts',(-2.58467719790652E-15,0.827002143027744,
-0.548473780018055));
#36273=CARTESIAN_POINT('Ctrl Pts',(-2.08860706507608E-15,0.8446799545592,
-0.50942695250173));
#36274=CARTESIAN_POINT('Ctrl Pts',(-1.61028094156565E-15,0.861725445715345,
-0.471776796999125));
#36275=CARTESIAN_POINT('Ctrl Pts',(-2.43875266999451E-15,0.876383418703462,
-0.433116863243482));
#36276=CARTESIAN_POINT('Ctrl Pts',(-2.39912256727592E-15,0.888437242092163,
-0.393609940259947));
#36277=CARTESIAN_POINT('Ctrl Pts',(-2.36446274816928E-15,0.898979312627847,
-0.359057852071011));
#36278=CARTESIAN_POINT('Ctrl Pts',(-1.01325357859657E-15,0.907528950391913,
-0.323857499715885));
#36279=CARTESIAN_POINT('Ctrl Pts',(-1.02695629777827E-15,0.913908649078052,
-0.288121577880467));
#36280=CARTESIAN_POINT('Ctrl Pts',(-0.0548926501499415,-1.2158567361346,
0.000987498914498598));
#36281=CARTESIAN_POINT('Ctrl Pts',(-0.0365951000999603,-1.21332229077892,
-0.308813117966906));
#36282=CARTESIAN_POINT('Ctrl Pts',(-0.0182975500499791,-1.08971454031158,
-0.620549786380947));
#36283=CARTESIAN_POINT('Ctrl Pts',(2.23779328401008E-15,-0.876385019502642,
-0.844404278593208));
#36284=CARTESIAN_POINT('',(-7.785,-0.556433207999828,-0.780144311992993));
#36285=CARTESIAN_POINT('Ctrl Pts',(-7.785,-0.5576340527839,-0.781217367305846));
#36286=CARTESIAN_POINT('Ctrl Pts',(-7.785,-0.578747991216662,-0.770087997067624));
#36287=CARTESIAN_POINT('Ctrl Pts',(-7.785,-0.5993761820992,-0.758139560309488));
#36288=CARTESIAN_POINT('Ctrl Pts',(-7.785,-0.619465300627149,-0.745383173566744));
#36289=CARTESIAN_POINT('Ctrl Pts',(-7.785,-0.655692140857232,-0.722379497034115));
#36290=CARTESIAN_POINT('Ctrl Pts',(-7.785,-0.690167491685533,-0.696752077864181));
#36291=CARTESIAN_POINT('Ctrl Pts',(-7.785,-0.722812205716661,-0.668816216966533));
#36292=CARTESIAN_POINT('Ctrl Pts',(-7.785,-0.7335642421842,-0.659615113387031));
#36293=CARTESIAN_POINT('Ctrl Pts',(-7.785,-0.744117533296352,-0.650163120371217));
#36294=CARTESIAN_POINT('Ctrl Pts',(-7.785,-0.754468725562236,-0.640470210083598));
#36295=CARTESIAN_POINT('Ctrl Pts',(-7.785,-0.763826437854487,-0.631707599611654));
#36296=CARTESIAN_POINT('Ctrl Pts',(-7.785,-0.773020919233301,-0.622745822047555));
#36297=CARTESIAN_POINT('Ctrl Pts',(-7.785,-0.782032296561331,-0.613610157430372));
#36298=CARTESIAN_POINT('Ctrl Pts',(-7.785,-0.812493295643311,-0.582729032227493));
#36299=CARTESIAN_POINT('Ctrl Pts',(-7.785,-0.840906423243611,-0.549826817131425));
#36300=CARTESIAN_POINT('Ctrl Pts',(-7.785,-0.867192555862543,-0.515209435590686));
#36301=CARTESIAN_POINT('Ctrl Pts',(-7.785,-0.884711533165385,-0.492137912278838));
#36302=CARTESIAN_POINT('Ctrl Pts',(-7.785,-0.901285379133529,-0.468303396752018));
#36303=CARTESIAN_POINT('Ctrl Pts',(-7.785,-0.916884395328298,-0.443785427125382));
#36304=CARTESIAN_POINT('Ctrl Pts',(-7.785,-0.922043717372295,-0.435676191287086));
#36305=CARTESIAN_POINT('Ctrl Pts',(-7.785,-0.927096351428236,-0.427492128011766));
#36306=CARTESIAN_POINT('Ctrl Pts',(-7.785,-0.932041071713118,-0.419235942078489));
#36307=CARTESIAN_POINT('Ctrl Pts',(-7.785,-0.93698833006316,-0.410975518344757));
#36308=CARTESIAN_POINT('Ctrl Pts',(-7.785,-0.941823150759485,-0.402650204861208));
#36309=CARTESIAN_POINT('Ctrl Pts',(-7.785,-0.946543129270692,-0.394266174047561));
#36310=CARTESIAN_POINT('Ctrl Pts',(-7.785,-0.969144618968524,-0.354119468800706));
#36311=CARTESIAN_POINT('Ctrl Pts',(-7.785,-0.989128076220463,-0.312608831398347));
#36312=CARTESIAN_POINT('Ctrl Pts',(-7.785,-1.0064033332032,-0.270063237970165));
#36313=CARTESIAN_POINT('Ctrl Pts',(-7.785,-1.02365060027322,-0.227586578245705));
#36314=CARTESIAN_POINT('Ctrl Pts',(-7.785,-1.03819918540846,-0.184077227350852));
#36315=CARTESIAN_POINT('Ctrl Pts',(-7.785,-1.04992333380568,-0.139823354894582));
#36316=CARTESIAN_POINT('Ctrl Pts',(-7.785,-1.05579967799946,-0.11764255526207));
#36317=CARTESIAN_POINT('Ctrl Pts',(-7.785,-1.06096583628138,-0.0952742038286101));
#36318=CARTESIAN_POINT('Ctrl Pts',(-7.785,-1.0654016453404,-0.0727521974605108));
#36319=CARTESIAN_POINT('Ctrl Pts',(-7.785,-1.06730690665633,-0.0630785828122528));
#36320=CARTESIAN_POINT('Ctrl Pts',(-7.785,-1.06907738892517,-0.0533766060944693));
#36321=CARTESIAN_POINT('Ctrl Pts',(-7.785,-1.07071130661907,-0.0436488970915968));
#36322=CARTESIAN_POINT('Ctrl Pts',(-7.785,-1.07200966230447,-0.0359189934759291));
#36323=CARTESIAN_POINT('Ctrl Pts',(-7.785,-1.07322141063688,-0.0281746421691217));
#36324=CARTESIAN_POINT('Ctrl Pts',(-7.785,-1.07434459151835,-0.0204264539147781));
#36325=CARTESIAN_POINT('Ctrl Pts',(-7.785,-1.0811257447752,0.0263528786774973));
#36326=CARTESIAN_POINT('Ctrl Pts',(-7.785,-1.08469796082786,0.0733627252990918));
#36327=CARTESIAN_POINT('Ctrl Pts',(-7.785,-1.08495012712384,0.120289602356072));
#36328=CARTESIAN_POINT('Ctrl Pts',(-7.785,-1.08497075310017,0.124127992620137));
#36329=CARTESIAN_POINT('Ctrl Pts',(-7.785,-1.08496914232922,0.127965843592304));
#36330=CARTESIAN_POINT('Ctrl Pts',(-7.785,-1.08494522067707,0.131802991509847));
#36331=CARTESIAN_POINT('Ctrl Pts',(-7.785,-1.08466326798781,0.177029557276298));
#36332=CARTESIAN_POINT('Ctrl Pts',(-7.785,-1.08128615140463,0.222157593215046));
#36333=CARTESIAN_POINT('Ctrl Pts',(-7.785,-1.07500410468562,0.266979872471771));
#36334=CARTESIAN_POINT('Ctrl Pts',(-7.785,-1.07185759882872,0.289430129610702));
#36335=CARTESIAN_POINT('Ctrl Pts',(-7.785,-1.06798150946743,0.311803845021642));
#36336=CARTESIAN_POINT('Ctrl Pts',(-7.785,-1.06339502635409,0.334075419501835));
#36337=CARTESIAN_POINT('Ctrl Pts',(-7.785,-1.06102777465901,0.345570593720789));
#36338=CARTESIAN_POINT('Ctrl Pts',(-7.785,-1.05847122649056,0.357038558179951));
#36339=CARTESIAN_POINT('Ctrl Pts',(-7.785,-1.05572770902942,0.368475774034161));
#36340=CARTESIAN_POINT('Ctrl Pts',(-7.785,-1.05326681078295,0.378734802758733));
#36341=CARTESIAN_POINT('Ctrl Pts',(-7.785,-1.0506549099214,0.388970584699868));
#36342=CARTESIAN_POINT('Ctrl Pts',(-7.785,-1.04789957705921,0.399160050513257));
#36343=CARTESIAN_POINT('Ctrl Pts',(-7.785,-1.0355261113626,0.44491822639059));
#36344=CARTESIAN_POINT('Ctrl Pts',(-7.785,-1.0202432411082,0.489835263872287));
#36345=CARTESIAN_POINT('Ctrl Pts',(-7.785,-1.00227600753725,0.533685063338825));
#36346=CARTESIAN_POINT('Ctrl Pts',(-7.785,-0.983902194037811,0.578527138453172));
#36347=CARTESIAN_POINT('Ctrl Pts',(-7.785,-0.962720954482079,0.622254138907397));
#36348=CARTESIAN_POINT('Ctrl Pts',(-7.785,-0.938918185991045,0.664625763107378));
#36349=CARTESIAN_POINT('Ctrl Pts',(-7.785,-0.926738910664416,0.686306252810178));
#36350=CARTESIAN_POINT('Ctrl Pts',(-7.785,-0.913872435977145,0.707631818960279));
#36351=CARTESIAN_POINT('Ctrl Pts',(-7.785,-0.900338597033089,0.728569055025174));
#36352=CARTESIAN_POINT('Ctrl Pts',(-7.785,-0.89089399903829,0.743180118343761));
#36353=CARTESIAN_POINT('Ctrl Pts',(-7.785,-0.88112432730713,0.75760204684153));
#36354=CARTESIAN_POINT('Ctrl Pts',(-7.785,-0.871035410752641,0.771823051085395));
#36355=CARTESIAN_POINT('Ctrl Pts',(-7.785,-0.865701397585292,0.77934170023667));
#36356=CARTESIAN_POINT('Ctrl Pts',(-7.785,-0.86027823994916,0.786803846419087));
#36357=CARTESIAN_POINT('Ctrl Pts',(-7.785,-0.854775425221195,0.794196577713452));
#36358=CARTESIAN_POINT('Ctrl Pts',(-7.785,-0.824631208231136,0.834693688247454));
#36359=CARTESIAN_POINT('Ctrl Pts',(-7.785,-0.792039562878693,0.873196157076302));
#36360=CARTESIAN_POINT('Ctrl Pts',(-7.785,-0.757211887306745,0.909454779884878));
#36361=CARTESIAN_POINT('Ctrl Pts',(-7.785,-0.722636821016273,0.945450414581139));
#36362=CARTESIAN_POINT('Ctrl Pts',(-7.785,-0.685857497318535,0.979235714907832));
#36363=CARTESIAN_POINT('Ctrl Pts',(-7.785,-0.647033561635485,1.01054947663034));
#36364=CARTESIAN_POINT('Ctrl Pts',(-7.785,-0.610160681532922,1.04028959857419));
#36365=CARTESIAN_POINT('Ctrl Pts',(-7.785,-0.571442820559113,1.06780104655221));
#36366=CARTESIAN_POINT('Ctrl Pts',(-7.785,-0.530983509300133,1.09283187766981));
#36367=CARTESIAN_POINT('Ctrl Pts',(-7.785,-0.557634052783907,-0.781217367305842));
#36368=CARTESIAN_POINT('Ctrl Pts',(-7.7629409778209,-0.31739492458004,-0.950718299157138));
#36369=CARTESIAN_POINT('Ctrl Pts',(-7.71705842806939,0.358267300689441,
-1.06099670633061));
#36370=CARTESIAN_POINT('Ctrl Pts',(-7.64735235074545,1.09209582283259,-0.300632258159738));
#36371=CARTESIAN_POINT('Ctrl Pts',(-7.5758817680282,0.844510306117659,0.755061250975084));
#36372=CARTESIAN_POINT('Ctrl Pts',(-7.50441118531095,-0.17668969425852,
1.11881329398577));
#36373=CARTESIAN_POINT('Ctrl Pts',(-7.44682637322301,-0.869040033824089,
0.586431559724317));
#36374=CARTESIAN_POINT('Ctrl Pts',(-7.41306508870749,-0.957373000383943,
0.133844055008089));
#36375=CARTESIAN_POINT('Ctrl Pts',(-7.40312733176438,-0.956848572177365,
0.000426154272836167));
#36376=CARTESIAN_POINT('Origin',(-7.785,-1.13809670924099E-16,0.));
#36377=CARTESIAN_POINT('',(-7.785,-1.215,-1.48794586096403E-16));
#36378=CARTESIAN_POINT('Origin',(-7.785,0.,0.));
#36379=CARTESIAN_POINT('Origin',(-7.785,0.,0.));
#36380=CARTESIAN_POINT('',(-7.785,0.556433207999845,-0.780144311992981));
#36381=CARTESIAN_POINT('Ctrl Pts',(-7.785,0.532258410758877,1.09442686519077));
#36382=CARTESIAN_POINT('Ctrl Pts',(-7.785,0.557739637633036,1.07882088466419));
#36383=CARTESIAN_POINT('Ctrl Pts',(-7.785,0.582563623672786,1.06223431603398));
#36384=CARTESIAN_POINT('Ctrl Pts',(-7.785,0.60666536531996,1.04466370008905));
#36385=CARTESIAN_POINT('Ctrl Pts',(-7.785,0.645212441942324,1.01656216746761));
#36386=CARTESIAN_POINT('Ctrl Pts',(-7.785,0.681913950695198,0.985944425966533));
#36387=CARTESIAN_POINT('Ctrl Pts',(-7.785,0.716645235920004,0.953067759411124));
#36388=CARTESIAN_POINT('Ctrl Pts',(-7.785,0.735328952881038,0.935381735742042));
#36389=CARTESIAN_POINT('Ctrl Pts',(-7.785,0.753441909891504,0.917041571835294));
#36390=CARTESIAN_POINT('Ctrl Pts',(-7.785,0.770960226206176,0.898085195601122));
#36391=CARTESIAN_POINT('Ctrl Pts',(-7.785,0.778530501447049,0.889893484532288));
#36392=CARTESIAN_POINT('Ctrl Pts',(-7.785,0.785989449819457,0.881586755557057));
#36393=CARTESIAN_POINT('Ctrl Pts',(-7.785,0.793326100456532,0.873178793404179));
#36394=CARTESIAN_POINT('Ctrl Pts',(-7.785,0.826126511808265,0.835588804336062));
#36395=CARTESIAN_POINT('Ctrl Pts',(-7.785,0.856535186295519,0.795925149890432));
#36396=CARTESIAN_POINT('Ctrl Pts',(-7.785,0.884405829267192,0.754483325808291));
#36397=CARTESIAN_POINT('Ctrl Pts',(-7.785,0.901804029846728,0.728613338937312));
#36398=CARTESIAN_POINT('Ctrl Pts',(-7.785,0.918212284704953,0.702049892369393));
#36399=CARTESIAN_POINT('Ctrl Pts',(-7.785,0.933585061142037,0.674862130976118));
#36400=CARTESIAN_POINT('Ctrl Pts',(-7.785,0.94077358376822,0.66214875816863));
#36401=CARTESIAN_POINT('Ctrl Pts',(-7.785,0.947735571875419,0.649298856397));
#36402=CARTESIAN_POINT('Ctrl Pts',(-7.785,0.95446575102645,0.63631947094407));
#36403=CARTESIAN_POINT('Ctrl Pts',(-7.785,0.958975356722034,0.627622538923361));
#36404=CARTESIAN_POINT('Ctrl Pts',(-7.785,0.96337845490693,0.61887200525621));
#36405=CARTESIAN_POINT('Ctrl Pts',(-7.785,0.967670436201489,0.610077271220812));
#36406=CARTESIAN_POINT('Ctrl Pts',(-7.785,0.988967668483222,0.566436938061539));
#36407=CARTESIAN_POINT('Ctrl Pts',(-7.785,1.00756077659699,0.521655942866011));
#36408=CARTESIAN_POINT('Ctrl Pts',(-7.785,1.02330935649198,0.476005300563686));
#36409=CARTESIAN_POINT('Ctrl Pts',(-7.785,1.0386172582705,0.431632058458665));
#36410=CARTESIAN_POINT('Ctrl Pts',(-7.785,1.05123767834139,0.386436094961105));
#36411=CARTESIAN_POINT('Ctrl Pts',(-7.785,1.06099323746147,0.340664258919277));
#36412=CARTESIAN_POINT('Ctrl Pts',(-7.785,1.06608164654541,0.316790094103385));
#36413=CARTESIAN_POINT('Ctrl Pts',(-7.785,1.07038983391497,0.292759321382559));
#36414=CARTESIAN_POINT('Ctrl Pts',(-7.785,1.07388705755652,0.268608144583126));
#36415=CARTESIAN_POINT('Ctrl Pts',(-7.785,1.07594738847747,0.254379881984722));
#36416=CARTESIAN_POINT('Ctrl Pts',(-7.785,1.07772617782379,0.240109850761259));
#36417=CARTESIAN_POINT('Ctrl Pts',(-7.785,1.07921648757224,0.225805690334931));
#36418=CARTESIAN_POINT('Ctrl Pts',(-7.785,1.08013730941692,0.216967538800246));
#36419=CARTESIAN_POINT('Ctrl Pts',(-7.785,1.08094784771634,0.208116602027595));
#36420=CARTESIAN_POINT('Ctrl Pts',(-7.785,1.08164565231098,0.199268521621097));
#36421=CARTESIAN_POINT('Ctrl Pts',(-7.785,1.08521244038656,0.154042067212324));
#36422=CARTESIAN_POINT('Ctrl Pts',(-7.785,1.08584829648986,0.108797261783825));
#36423=CARTESIAN_POINT('Ctrl Pts',(-7.785,1.08340106664489,0.0637641771385276));
#36424=CARTESIAN_POINT('Ctrl Pts',(-7.785,1.08315610349527,0.0592564492377615));
#36425=CARTESIAN_POINT('Ctrl Pts',(-7.785,1.08288020632508,0.0547508504375447));
#36426=CARTESIAN_POINT('Ctrl Pts',(-7.785,1.08257319383316,0.0502476177093405));
#36427=CARTESIAN_POINT('Ctrl Pts',(-7.785,1.07966075959026,0.00752828365533442));
#36428=CARTESIAN_POINT('Ctrl Pts',(-7.785,1.07395105666554,-0.0349795970626121));
#36429=CARTESIAN_POINT('Ctrl Pts',(-7.785,1.06556613520383,-0.0770620868862156));
#36430=CARTESIAN_POINT('Ctrl Pts',(-7.785,1.06139056925744,-0.0980185397580686));
#36431=CARTESIAN_POINT('Ctrl Pts',(-7.785,1.05655104212579,-0.118869222739669));
#36432=CARTESIAN_POINT('Ctrl Pts',(-7.785,1.05105978648461,-0.139585623514728));
#36433=CARTESIAN_POINT('Ctrl Pts',(-7.785,1.04643720856273,-0.157024836529205));
#36434=CARTESIAN_POINT('Ctrl Pts',(-7.785,1.04135275390333,-0.174368872848005));
#36435=CARTESIAN_POINT('Ctrl Pts',(-7.785,1.03581286032973,-0.191599736380545));
#36436=CARTESIAN_POINT('Ctrl Pts',(-7.785,1.03314821815863,-0.199887636681043));
#36437=CARTESIAN_POINT('Ctrl Pts',(-7.785,1.0303812524574,-0.208139819618536));
#36438=CARTESIAN_POINT('Ctrl Pts',(-7.785,1.02751360825937,-0.216353690840345));
#36439=CARTESIAN_POINT('Ctrl Pts',(-7.785,1.01263586389863,-0.258968418404492));
#36440=CARTESIAN_POINT('Ctrl Pts',(-7.785,0.995049070732015,-0.300562539231134));
#36441=CARTESIAN_POINT('Ctrl Pts',(-7.785,0.97491261572845,-0.340890293089778));
#36442=CARTESIAN_POINT('Ctrl Pts',(-7.785,0.954937271641593,-0.380895386311694));
#36443=CARTESIAN_POINT('Ctrl Pts',(-7.785,0.9324520326871,-0.419655189247156));
#36444=CARTESIAN_POINT('Ctrl Pts',(-7.785,0.907576185682416,-0.456894436402826));
#36445=CARTESIAN_POINT('Ctrl Pts',(-7.785,0.896398825208152,-0.473626991847904));
#36446=CARTESIAN_POINT('Ctrl Pts',(-7.785,0.884738404704367,-0.490051998613649));
#36447=CARTESIAN_POINT('Ctrl Pts',(-7.785,0.872604028769965,-0.506141415467363));
#36448=CARTESIAN_POINT('Ctrl Pts',(-7.785,0.865105828753884,-0.516083555579341));
#36449=CARTESIAN_POINT('Ctrl Pts',(-7.785,0.857426636030853,-0.525897514492815));
#36450=CARTESIAN_POINT('Ctrl Pts',(-7.785,0.84956844738637,-0.535576253967916));
#36451=CARTESIAN_POINT('Ctrl Pts',(-7.785,0.844755476884386,-0.541504272458888));
#36452=CARTESIAN_POINT('Ctrl Pts',(-7.785,0.839876635612896,-0.547379881046622));
#36453=CARTESIAN_POINT('Ctrl Pts',(-7.785,0.834938380506431,-0.553194836113957));
#36454=CARTESIAN_POINT('Ctrl Pts',(-7.785,0.807036952950441,-0.586049669259403));
#36455=CARTESIAN_POINT('Ctrl Pts',(-7.785,0.777189661728921,-0.617035617704938));
#36456=CARTESIAN_POINT('Ctrl Pts',(-7.785,0.745516763485908,-0.645914476150201));
#36457=CARTESIAN_POINT('Ctrl Pts',(-7.785,0.714976782555787,-0.673760358122703));
#36458=CARTESIAN_POINT('Ctrl Pts',(-7.785,0.682738657926675,-0.699647618275338));
#36459=CARTESIAN_POINT('Ctrl Pts',(-7.785,0.648890268218106,-0.723319923617524));
#36460=CARTESIAN_POINT('Ctrl Pts',(-7.785,0.619286115682046,-0.744023967274078));
#36461=CARTESIAN_POINT('Ctrl Pts',(-7.785,0.588449651909176,-0.763033317509813));
#36462=CARTESIAN_POINT('Ctrl Pts',(-7.785,0.556433207999864,-0.780144311992967));
#36463=CARTESIAN_POINT('Origin',(-7.785,0.,0.));
#36464=CARTESIAN_POINT('Origin',(-8.61687266823562,0.,0.));
#36465=CARTESIAN_POINT('Ctrl Pts',(-7.785,0.556433207999845,-0.780144311992981));
#36466=CARTESIAN_POINT('Ctrl Pts',(-7.76117647242759,0.815939785066093,
-0.595052816798781));
#36467=CARTESIAN_POINT('Ctrl Pts',(-7.71352941728275,1.13124973052358,0.0512203649262202));
#36468=CARTESIAN_POINT('Ctrl Pts',(-7.64205883456552,0.569045812913815,
0.980302233127841));
#36469=CARTESIAN_POINT('Ctrl Pts',(-7.57058825184826,-0.514804186274824,
1.00861045471588));
#36470=CARTESIAN_POINT('Ctrl Pts',(-7.52052619640497,-0.943555255514336,
0.382401100605641));
#36471=CARTESIAN_POINT('Ctrl Pts',(-7.49428766853409,-0.959633789666665,
0.0328156789457131));
#36472=CARTESIAN_POINT('Ctrl Pts',(-7.49187266823563,-0.959412934693052,
0.000617836956614886));
#36473=CARTESIAN_POINT('Ctrl Pts',(-7.93323468161444,0.705521886480338,
-0.989173325407244));
#36474=CARTESIAN_POINT('Ctrl Pts',(-7.90941115404203,1.03455970660609,-0.754489092001615));
#36475=CARTESIAN_POINT('Ctrl Pts',(-7.8617640988972,1.43435264553733,0.0649441621553011));
#36476=CARTESIAN_POINT('Ctrl Pts',(-7.79029351617995,0.721513866621781,
1.24296082781143));
#36477=CARTESIAN_POINT('Ctrl Pts',(-7.7188229334627,-0.652738936941171,
1.27885385074857));
#36478=CARTESIAN_POINT('Ctrl Pts',(-7.64735235074546,-1.42884542185819,
0.145316990997596));
#36479=CARTESIAN_POINT('Ctrl Pts',(-7.5758817680282,-0.896443945405535,
-1.12228602947411));
#36480=CARTESIAN_POINT('Ctrl Pts',(-7.50441118531097,0.457089628791888,
-1.36148449659785));
#36481=CARTESIAN_POINT('Ctrl Pts',(-7.4329406025937,1.3919330456215,-0.353977390791757));
#36482=CARTESIAN_POINT('Ctrl Pts',(-7.36147001987648,1.05193816003137,0.977876750342409));
#36483=CARTESIAN_POINT('Ctrl Pts',(-7.28999943715921,-0.25153214713002,
1.41402569308405));
#36484=CARTESIAN_POINT('Ctrl Pts',(-7.21852885444197,-1.32461931868978,
0.555117463789919));
#36485=CARTESIAN_POINT('Ctrl Pts',(-7.14705827172472,-1.18450017731315,
-0.81223974728715));
#36486=CARTESIAN_POINT('Ctrl Pts',(-7.07558768900747,0.0404963929544019,
-1.43566122947319));
#36487=CARTESIAN_POINT('Ctrl Pts',(-7.00411710629023,1.22840163452736,-0.744176158150377));
#36488=CARTESIAN_POINT('Ctrl Pts',(-6.93264652357298,1.29122272974647,0.628897789905487));
#36489=CARTESIAN_POINT('Ctrl Pts',(-6.86117594085574,0.171421495630961,
1.42596696158188));
#36490=CARTESIAN_POINT('Ctrl Pts',(-6.78970535813848,-1.10538337312329,
0.917003589837982));
#36491=CARTESIAN_POINT('Ctrl Pts',(-6.71823477542124,-1.36977524784193,
-0.431837537599902));
#36492=CARTESIAN_POINT('Ctrl Pts',(-6.64676419270399,-0.379599306735098,
-1.38516138616941));
#36493=CARTESIAN_POINT('Ctrl Pts',(-6.57529360998674,0.958249021520171,
-1.06982552176842));
#36494=CARTESIAN_POINT('Ctrl Pts',(-6.5038230272695,1.41844363852531,0.225356282468531));
#36495=CARTESIAN_POINT('Ctrl Pts',(-6.43235244455225,0.579495426924149,
1.31413577551544));
#36496=CARTESIAN_POINT('Ctrl Pts',(-6.360881861835,-0.790208678038612,1.19930732160193));
#36497=CARTESIAN_POINT('Ctrl Pts',(-6.28941127911776,-1.43616606331737,
-0.0139585114361597));
#36498=CARTESIAN_POINT('Ctrl Pts',(-6.2179406964005,-0.766748777246146,
-1.21443983438033));
#36499=CARTESIAN_POINT('Ctrl Pts',(-6.14647011368326,0.60492846703713,-1.30262402536569));
#36500=CARTESIAN_POINT('Ctrl Pts',(-6.07499953096601,1.42255586777629,-0.197743783258168));
#36501=CARTESIAN_POINT('Ctrl Pts',(-6.00352894824877,0.937274082844972,
1.08824863615832));
#36502=CARTESIAN_POINT('Ctrl Pts',(-5.93205836553151,-0.406450621262066,
1.37752157637255));
#36503=CARTESIAN_POINT('Ctrl Pts',(-5.86058778281429,-1.37790998250129,
0.405131930188321));
#36504=CARTESIAN_POINT('Ctrl Pts',(-5.789117200097,-1.08735101901064,-0.93831527865966));
#36505=CARTESIAN_POINT('Ctrl Pts',(-5.71764661737979,0.199105302652743,
-1.42236594420155));
#36506=CARTESIAN_POINT('Ctrl Pts',(-5.64617603466251,1.3032024399867,-0.603681373867629));
#36507=CARTESIAN_POINT('Ctrl Pts',(-5.57470545194529,1.21370537961352,0.767910836124945));
#36508=CARTESIAN_POINT('Ctrl Pts',(-5.50323486922803,0.0125838667550361,
1.43617876569961));
#36509=CARTESIAN_POINT('Ctrl Pts',(-5.43176428651079,-1.2000631235608,0.789060390726951));
#36510=CARTESIAN_POINT('Ctrl Pts',(-5.36029370379354,-1.31358051036201,
-0.580752997015039));
#36511=CARTESIAN_POINT('Ctrl Pts',(-5.28882312107629,-0.223998495813416,
-1.41865868855736));
#36512=CARTESIAN_POINT('Ctrl Pts',(-5.21735253835905,1.07074220835543,-0.957224594330622));
#36513=CARTESIAN_POINT('Ctrl Pts',(-5.1458819556418,1.3847974503765,0.380924956095192));
#36514=CARTESIAN_POINT('Ctrl Pts',(-5.07441137292455,0.430526182985665,
1.37018794568822));
#36515=CARTESIAN_POINT('Ctrl Pts',(-5.00294079020731,-0.918061069553906,
1.10450517124862));
#36516=CARTESIAN_POINT('Ctrl Pts',(-4.93147020749005,-1.42580247026315,
-0.172786332031617));
#36517=CARTESIAN_POINT('Ctrl Pts',(-4.85999962477281,-0.627661144420497,
-1.29182401608353));
#36518=CARTESIAN_POINT('Ctrl Pts',(-4.78852904205556,0.745350728865686,
-1.22768892302766));
#36519=CARTESIAN_POINT('Ctrl Pts',(-4.71705845933832,1.43570096959843,-0.0391219457536234));
#36520=CARTESIAN_POINT('Ctrl Pts',(-4.64558787662107,0.811102515967952,
1.18527655394675));
#36521=CARTESIAN_POINT('Ctrl Pts',(-4.57411729390382,-0.556379182120533,
1.32408836806624));
#36522=CARTESIAN_POINT('Ctrl Pts',(-4.50264671118658,-1.41427699429376,
0.250176705863753));
#36523=CARTESIAN_POINT('Ctrl Pts',(-4.43117612846932,-0.976848184493127,
-1.05287008942125));
#36524=CARTESIAN_POINT('Ctrl Pts',(-4.35970554575208,0.355269193463592,
-1.39160037400151));
#36525=CARTESIAN_POINT('Ctrl Pts',(-4.28823496303483,1.36199794803372,-0.455773397970269));
#36526=CARTESIAN_POINT('Ctrl Pts',(-4.21676438031759,1.12128210138353,0.897493314661654));
#36527=CARTESIAN_POINT('Ctrl Pts',(-4.14529379760033,-0.146408349622836,
1.42875204143551));
#36528=CARTESIAN_POINT('Ctrl Pts',(-4.07382321488309,-1.28000439499941,
0.651426549602967));
#36529=CARTESIAN_POINT('Ctrl Pts',(-4.00235263216585,-1.24125317334416,
-0.722536061666472));
#36530=CARTESIAN_POINT('Ctrl Pts',(-3.93088204944859,-0.06564666341837,
-1.43473283796234));
#36531=CARTESIAN_POINT('Ctrl Pts',(-3.85941146673135,1.17008517634921,-0.832867625036097));
#36532=CARTESIAN_POINT('Ctrl Pts',(-3.78794088401411,1.33414400933146,0.531815346817302));
#36533=CARTESIAN_POINT('Ctrl Pts',(-3.71647030129685,0.276269472961998,
1.40941228143319));
#36534=CARTESIAN_POINT('Ctrl Pts',(-3.64499971857961,-1.03463838333717,
0.996138151297738));
#36535=CARTESIAN_POINT('Ctrl Pts',(-3.57352913586236,-1.39792802378473,
-0.329492095599789));
#36536=CARTESIAN_POINT('Ctrl Pts',(-3.50205855314511,-0.480864952480873,
-1.35334278666603));
#36537=CARTESIAN_POINT('Ctrl Pts',(-3.43058797042787,0.876619038512565,
-1.13767607958625));
#36538=CARTESIAN_POINT('Ctrl Pts',(-3.35911738771062,1.431213650342,0.119980364310839));
#36539=CARTESIAN_POINT('Ctrl Pts',(-3.28764680499337,0.674969472810977,
1.2677476134936));
#36540=CARTESIAN_POINT('Ctrl Pts',(-3.21617622227613,-0.699474626432212,
1.25439349795945));
#36541=CARTESIAN_POINT('Ctrl Pts',(-3.14470563955887,-1.43327470143649,
0.0921489607514472));
#36542=CARTESIAN_POINT('Ctrl Pts',(-3.07323505684163,-0.854348284485474,
-1.15449417908544));
#36543=CARTESIAN_POINT('Ctrl Pts',(-3.00176447412438,0.507069880402349,
-1.34374399985048));
#36544=CARTESIAN_POINT('Ctrl Pts',(-2.93029389140714,1.40406621142284,-0.302267885634783));
#36545=CARTESIAN_POINT('Ctrl Pts',(-2.85882330868989,1.01508790663436,1.01605331678519));
#36546=CARTESIAN_POINT('Ctrl Pts',(-2.78735272597264,-0.303602466166582,
1.40377823864132));
#36547=CARTESIAN_POINT('Ctrl Pts',(-2.71588214325539,-1.34422541758585,
0.505792276988717));
#36548=CARTESIAN_POINT('Ctrl Pts',(-2.64441156053815,-1.15368150681488,
-0.855445370306784));
#36549=CARTESIAN_POINT('Ctrl Pts',(-2.5729409778209,0.0935114020565075,
-1.4331864562681));
#36550=CARTESIAN_POINT('Ctrl Pts',(-2.50147039510365,1.25505785762914,-0.698281873420766));
#36551=CARTESIAN_POINT('Ctrl Pts',(-2.4299998123864,1.26710540905413,0.676174299345015));
#36552=CARTESIAN_POINT('Ctrl Pts',(-2.35852922966916,0.118619786410601,
1.43132705801742));
#36553=CARTESIAN_POINT('Ctrl Pts',(-2.28705864695191,-1.13850888695148,
0.875537158020446));
#36554=CARTESIAN_POINT('Ctrl Pts',(-2.21558806423466,-1.35288506094146,
-0.482151234210018));
#36555=CARTESIAN_POINT('Ctrl Pts',(-2.14411748151742,-0.328163064620681,
-1.39824061009842));
#36556=CARTESIAN_POINT('Ctrl Pts',(-2.07264689880017,0.997121237106055,
-1.03369097860381));
#36557=CARTESIAN_POINT('Ctrl Pts',(-2.00117631608292,1.40914902059169,0.277609147294719));
#36558=CARTESIAN_POINT('Ctrl Pts',(-1.92970573336567,0.530546857965926,
1.33464895458537));
#36559=CARTESIAN_POINT('Ctrl Pts',(-1.85823515064843,-0.833979541327682,
1.16929291685568));
#36560=CARTESIAN_POINT('Ctrl Pts',(-1.78676456793118,-1.43466978575981,
-0.0670105030551046));
#36561=CARTESIAN_POINT('Ctrl Pts',(-1.71529398521393,-0.72135578893274,
-1.24193946088825));
#36562=CARTESIAN_POINT('Ctrl Pts',(-1.64382340249668,0.652643037024826,
-1.27938456598828));
#36563=CARTESIAN_POINT('Ctrl Pts',(-1.57235281977944,1.42889057506806,-0.145050098163382));
#36564=CARTESIAN_POINT('Ctrl Pts',(-1.50088223706219,0.896427004851561,
1.12213475629642));
#36565=CARTESIAN_POINT('Ctrl Pts',(-1.42941165434495,-0.457067910847659,
1.36156407656574));
#36566=CARTESIAN_POINT('Ctrl Pts',(-1.3579410716277,-1.39193748201553,0.353946154706768));
#36567=CARTESIAN_POINT('Ctrl Pts',(-1.28647048891045,-1.05194098533954,
-0.977848588878373));
#36568=CARTESIAN_POINT('Ctrl Pts',(-1.2149999061932,0.25152096267351,-1.414038575788));
#36569=CARTESIAN_POINT('Ctrl Pts',(-1.14352932347596,1.32461677048183,-0.555120164209031));
#36570=CARTESIAN_POINT('Ctrl Pts',(-1.07205874075871,1.18450478400261,0.812228737094626));
#36571=CARTESIAN_POINT('Ctrl Pts',(-1.00058815804146,-0.0404863500284713,
1.43566340881953));
#36572=CARTESIAN_POINT('Ctrl Pts',(-0.929117575324211,-1.22839760243372,
0.744182813832753));
#36573=CARTESIAN_POINT('Ctrl Pts',(-0.857646992606967,-1.29122544848478,
-0.628887879387163));
#36574=CARTESIAN_POINT('Ctrl Pts',(-0.786176409889718,-0.171433387447648,
-1.42596797677794));
#36575=CARTESIAN_POINT('Ctrl Pts',(-0.714705827172472,1.1053821595978,-0.917007098824021));
#36576=CARTESIAN_POINT('Ctrl Pts',(-0.643235244455224,1.36976900842759,
0.431821659129023));
#36577=CARTESIAN_POINT('Ctrl Pts',(-0.571764661737977,0.379625575419958,
1.38517192213728));
#36578=CARTESIAN_POINT('Ctrl Pts',(-0.500294079020729,-0.958274652820194,
1.06980712581625));
#36579=CARTESIAN_POINT('Ctrl Pts',(-0.428823496303483,-1.41838316065648,
-0.225300183736171));
#36580=CARTESIAN_POINT('Ctrl Pts',(-0.357352913586234,-0.579621661001341,
-1.31422083734243));
#36581=CARTESIAN_POINT('Ctrl Pts',(-0.285882330868989,0.790424325774726,
-1.19914371643322));
#36582=CARTESIAN_POINT('Ctrl Pts',(-0.21441174815174,1.43574007932854,0.0136277651574338));
#36583=CARTESIAN_POINT('Ctrl Pts',(-0.142941165434494,0.767580850576639,
1.21505288651533));
#36584=CARTESIAN_POINT('Ctrl Pts',(-0.0714705827172464,-0.606613081372982,
1.30138611697881));
#36585=CARTESIAN_POINT('Ctrl Pts',(-0.0238235275724144,-1.14778002846286,
0.567598962951908));
#36586=CARTESIAN_POINT('Ctrl Pts',(1.11022302462516E-15,-1.20342780657953,
0.167291704370495));
#36587=CARTESIAN_POINT('Ctrl Pts',(-7.8838231210763,0.655825660320174,-0.919496987602489));
#36588=CARTESIAN_POINT('Ctrl Pts',(-7.85999959350388,0.961686399426088,
-0.701343666934003));
#36589=CARTESIAN_POINT('Ctrl Pts',(-7.81235253835904,1.33331834053275,0.0603695630789417));
#36590=CARTESIAN_POINT('Ctrl Pts',(-7.74088195564181,0.670691182052459,
1.1554079629169));
#36591=CARTESIAN_POINT('Ctrl Pts',(-7.66941137292454,-0.606760686719055,
1.18877271873767));
#36592=CARTESIAN_POINT('Ctrl Pts',(-7.59794079020731,-1.32819903994816,
0.135081013648165));
#36593=CARTESIAN_POINT('Ctrl Pts',(-7.52647020749005,-0.833299368455494,
-1.04323337156808));
#36594=CARTESIAN_POINT('Ctrl Pts',(-7.45499962477282,0.424892711866708,
-1.26558294803777));
#36595=CARTESIAN_POINT('Ctrl Pts',(-7.38352904205555,1.29388673301154,-0.329043592414301));
#36596=CARTESIAN_POINT('Ctrl Pts',(-7.31205845933833,0.977840732709539,
0.908996131508284));
#36597=CARTESIAN_POINT('Ctrl Pts',(-7.24058787662107,-0.233814484914493,
1.31442319741893));
#36598=CARTESIAN_POINT('Ctrl Pts',(-7.16911729390383,-1.23131451482871,
0.51601556836383));
#36599=CARTESIAN_POINT('Ctrl Pts',(-7.09764671118657,-1.10106521969307,
-0.755026426267688));
#36600=CARTESIAN_POINT('Ctrl Pts',(-7.02617612846933,0.0376438692531656,
-1.3345347491804));
#36601=CARTESIAN_POINT('Ctrl Pts',(-6.95470554575208,1.14187430402945,-0.691757165391766));
#36602=CARTESIAN_POINT('Ctrl Pts',(-6.88323496303484,1.20027034679381,0.584598885225599));
#36603=CARTESIAN_POINT('Ctrl Pts',(-6.81176438031758,0.159346744189729,
1.32552333541284));
#36604=CARTESIAN_POINT('Ctrl Pts',(-6.74029379760034,-1.0275213207092,0.852410812968044));
#36605=CARTESIAN_POINT('Ctrl Pts',(-6.66882321488309,-1.27328970740752,
-0.401419351652376));
#36606=CARTESIAN_POINT('Ctrl Pts',(-6.59735263216585,-0.352860727310056,
-1.28759206219164));
#36607=CARTESIAN_POINT('Ctrl Pts',(-6.5258820494486,0.890750959441906,-0.994468127333838));
#36608=CARTESIAN_POINT('Ctrl Pts',(-6.45441146673135,1.31852994738913,0.209482420870793));
#36609=CARTESIAN_POINT('Ctrl Pts',(-6.38294088401411,0.538676373189495,
1.22156942150623));
#36610=CARTESIAN_POINT('Ctrl Pts',(-6.31147030129686,-0.734547202569097,
1.11482936417495));
#36611=CARTESIAN_POINT('Ctrl Pts',(-6.23999971857961,-1.33500402305489,
-0.0129752884426916));
#36612=CARTESIAN_POINT('Ctrl Pts',(-6.16852913586237,-0.712739792730926,
-1.12889595852926));
#36613=CARTESIAN_POINT('Ctrl Pts',(-6.09705855314511,0.562317936471494,
-1.21086854703574));
#36614=CARTESIAN_POINT('Ctrl Pts',(-6.02558797042787,1.32235251549876,-0.183814917318094));
#36615=CARTESIAN_POINT('Ctrl Pts',(-5.95411738771061,0.871253473580096,
1.01159353675267));
#36616=CARTESIAN_POINT('Ctrl Pts',(-5.88264680499337,-0.377820663234907,
1.28049039263217));
#36617=CARTESIAN_POINT('Ctrl Pts',(-5.81117622227613,-1.28085143983814,
0.376594859385609));
#36618=CARTESIAN_POINT('Ctrl Pts',(-5.73970563955887,-1.01075914682107,
-0.872221328647086));
#36619=CARTESIAN_POINT('Ctrl Pts',(-5.66823505684163,0.185080532705953,
-1.32217596994263));
#36620=CARTESIAN_POINT('Ctrl Pts',(-5.59676447412438,1.21140621873387,-0.561158687244707));
#36621=CARTESIAN_POINT('Ctrl Pts',(-5.52529389140713,1.12821323799053,0.713819997393794));
#36622=CARTESIAN_POINT('Ctrl Pts',(-5.45382330868989,0.0116974722997823,
1.33501583069457));
#36623=CARTESIAN_POINT('Ctrl Pts',(-5.38235272597264,-1.11553192823179,
0.733479799418535));
#36624=CARTESIAN_POINT('Ctrl Pts',(-5.3108821432554,-1.22105326865133,-0.539845361354251));
#36625=CARTESIAN_POINT('Ctrl Pts',(-5.23941156053815,-0.208220275292116,
-1.31872984952112));
#36626=CARTESIAN_POINT('Ctrl Pts',(-5.1679409778209,0.995320243473335,-0.889798691835582));
#36627=CARTESIAN_POINT('Ctrl Pts',(-5.09647039510366,1.28725376165656,0.354092999311268));
#36628=CARTESIAN_POINT('Ctrl Pts',(-5.0249998123864,0.400200367490025,1.27367333524777));
#36629=CARTESIAN_POINT('Ctrl Pts',(-4.95352922966917,-0.853393804915241,
1.02670497845901));
#36630=CARTESIAN_POINT('Ctrl Pts',(-4.8820586469519,-1.32537043069111,-0.16061544293722));
#36631=CARTESIAN_POINT('Ctrl Pts',(-4.81058806423467,-0.583449347759317,
-1.20082927914816));
#36632=CARTESIAN_POINT('Ctrl Pts',(-4.73911748151741,0.692849000570423,
-1.14121179518476));
#36633=CARTESIAN_POINT('Ctrl Pts',(-4.66764689880018,1.33457169005264,-0.0363662366802944));
#36634=CARTESIAN_POINT('Ctrl Pts',(-4.59617631608292,0.753969300337004,
1.10178690916601));
#36635=CARTESIAN_POINT('Ctrl Pts',(-4.52470573336568,-0.517188412570627,
1.23082096381356));
#36636=CARTESIAN_POINT('Ctrl Pts',(-4.45323515064843,-1.31465679723343,
0.232554519517921));
#36637=CARTESIAN_POINT('Ctrl Pts',(-4.38176456793118,-0.908040016765106,
-0.978707017964768));
#36638=CARTESIAN_POINT('Ctrl Pts',(-4.31029398521394,0.33024440185269,-1.29357749443364));
#36639=CARTESIAN_POINT('Ctrl Pts',(-4.23882340249668,1.26606023248978,-0.423669194971941));
#36640=CARTESIAN_POINT('Ctrl Pts',(-4.16735281977945,1.04230015912558,0.834274821235221));
#36641=CARTESIAN_POINT('Ctrl Pts',(-4.09588223706219,-0.136095498109634,
1.3281122371451));
#36642=CARTESIAN_POINT('Ctrl Pts',(-4.02441165434495,-1.18984221985096,
0.60554074257674));
#36643=CARTESIAN_POINT('Ctrl Pts',(-3.9529410716277,-1.15382059385002,-0.671641374743884));
#36644=CARTESIAN_POINT('Ctrl Pts',(-3.88147048891045,-0.0610225808853908,
-1.33367175259969));
#36645=CARTESIAN_POINT('Ctrl Pts',(-3.8099999061932,1.08766559636906,-0.774201297813038));
#36646=CARTESIAN_POINT('Ctrl Pts',(-3.73852932347596,1.24016829619131,0.494354828217767));
#36647=CARTESIAN_POINT('Ctrl Pts',(-3.66705874075871,0.256809339304101,
1.31013474967518));
#36648=CARTESIAN_POINT('Ctrl Pts',(-3.59558815804146,-0.961759534250261,
0.925971218418253));
#36649=CARTESIAN_POINT('Ctrl Pts',(-3.52411757532421,-1.29945943116285,
-0.306283015889169));
#36650=CARTESIAN_POINT('Ctrl Pts',(-3.45264699260697,-0.446993326541367,
-1.25801473166563));
#36651=CARTESIAN_POINT('Ctrl Pts',(-3.38117640988971,0.814870907336141,
-1.05753936259481));
#36652=CARTESIAN_POINT('Ctrl Pts',(-3.30970582717248,1.33040045288649,0.111529072531204));
#36653=CARTESIAN_POINT('Ctrl Pts',(-3.23823524445522,0.627425326818042,
1.17844879325643));
#36654=CARTESIAN_POINT('Ctrl Pts',(-3.16676466173798,-0.650204362965427,
1.16603532769852));
#36655=CARTESIAN_POINT('Ctrl Pts',(-3.09529407902073,-1.33231632569059,
0.0856580840236087));
#36656=CARTESIAN_POINT('Ctrl Pts',(-3.02382349630348,-0.794168882004904,
-1.07317281269857));
#36657=CARTESIAN_POINT('Ctrl Pts',(-2.95235291358624,0.47135240665934,-1.24909207338638));
#36658=CARTESIAN_POINT('Ctrl Pts',(-2.88088233086899,1.30516525126295,-0.280976450892185));
#36659=CARTESIAN_POINT('Ctrl Pts',(-2.80941174815174,0.943586172744538,
0.94448358041082));
#36660=CARTESIAN_POINT('Ctrl Pts',(-2.7379411654345,-0.282217024962677,
1.30489756298394));
#36661=CARTESIAN_POINT('Ctrl Pts',(-2.66647058271725,-1.24953958055837,
0.470164796298212));
#36662=CARTESIAN_POINT('Ctrl Pts',(-2.595,-1.0724173842155,-0.795188690244717));
#36663=CARTESIAN_POINT('Ctrl Pts',(-2.52352941728275,0.0869245563835385,
-1.33223429641986));
#36664=CARTESIAN_POINT('Ctrl Pts',(-2.45205883456551,1.1666528905657,-0.649095626232613));
#36665=CARTESIAN_POINT('Ctrl Pts',(-2.38058825184826,1.17785182502816,0.628545286627099));
#36666=CARTESIAN_POINT('Ctrl Pts',(-2.30911766913101,0.110264332319804,
1.33050587224349));
#36667=CARTESIAN_POINT('Ctrl Pts',(-2.23764708641377,-1.05831350787747,
0.813865233377982));
#36668=CARTESIAN_POINT('Ctrl Pts',(-2.16617650369651,-1.25758924766389,
-0.448189003926511));
#36669=CARTESIAN_POINT('Ctrl Pts',(-2.09470592097927,-0.305047600466661,
-1.29974999922249));
#36670=CARTESIAN_POINT('Ctrl Pts',(-2.02323533826202,0.926885056687137,
-0.960878863718607));
#36671=CARTESIAN_POINT('Ctrl Pts',(-1.95176475554478,1.30989003265289,0.25805464837349));
#36672=CARTESIAN_POINT('Ctrl Pts',(-1.88029417282753,0.493175690398631,
1.24063767362796));
#36673=CARTESIAN_POINT('Ctrl Pts',(-1.80882359011028,-0.775234891880261,
1.0869291428083));
#36674=CARTESIAN_POINT('Ctrl Pts',(-1.73735300739303,-1.33361314172858,
-0.0622903530799726));
#36675=CARTESIAN_POINT('Ctrl Pts',(-1.66588242467579,-0.670544239191035,
-1.15445854001498));
#36676=CARTESIAN_POINT('Ctrl Pts',(-1.59441184195854,0.606671541892842,
-1.18926605094919));
#36677=CARTESIAN_POINT('Ctrl Pts',(-1.52294125924129,1.32824101261299,-0.13483292046695));
#36678=CARTESIAN_POINT('Ctrl Pts',(-1.45147067652404,0.83328362117648,1.04309275391532));
#36679=CARTESIAN_POINT('Ctrl Pts',(-1.3800000938068,-0.424872523711829,
1.26565692247568));
#36680=CARTESIAN_POINT('Ctrl Pts',(-1.30852951108955,-1.2938908569106,0.329014556566575));
#36681=CARTESIAN_POINT('Ctrl Pts',(-1.23705892837231,-0.97784335900594,
-0.908969953708416));
#36682=CARTESIAN_POINT('Ctrl Pts',(-1.16558834565505,0.23380408827944,-1.31443517267865));
#36683=CARTESIAN_POINT('Ctrl Pts',(-1.09411776293781,1.23131214611387,-0.516018078568234));
#36684=CARTESIAN_POINT('Ctrl Pts',(-1.02264718022056,1.10106950189213,0.755016191621646));
#36685=CARTESIAN_POINT('Ctrl Pts',(-0.951176597503315,-0.0376345337404676,
1.33453677501585));
#36686=CARTESIAN_POINT('Ctrl Pts',(-0.879706014786067,-1.14187055595229,
0.691763352254813));
#36687=CARTESIAN_POINT('Ctrl Pts',(-0.808235432068821,-1.20027287402703,
-0.584589672793852));
#36688=CARTESIAN_POINT('Ctrl Pts',(-0.736764849351572,-0.159357798359248,
-1.32552427909955));
#36689=CARTESIAN_POINT('Ctrl Pts',(-0.665294266634327,1.02752019266317,
-0.852414074784762));
#36690=CARTESIAN_POINT('Ctrl Pts',(-0.593823683917078,1.27328390749102,
0.401404591644431));
#36691=CARTESIAN_POINT('Ctrl Pts',(-0.522353101199832,0.352885145656143,
1.28760185601691));
#36692=CARTESIAN_POINT('Ctrl Pts',(-0.450882518482584,-0.890774785299878,
0.994451027173357));
#36693=CARTESIAN_POINT('Ctrl Pts',(-0.379411935765338,-1.31847372951833,
-0.209430273674656));
#36694=CARTESIAN_POINT('Ctrl Pts',(-0.307941353048089,-0.538793715469893,
-1.22164849166681));
#36695=CARTESIAN_POINT('Ctrl Pts',(-0.236470770330843,0.734747660303497,
-1.11467728318377));
#36696=CARTESIAN_POINT('Ctrl Pts',(-0.165000187613595,1.33460804493414,
0.0126678395870271));
#36697=CARTESIAN_POINT('Ctrl Pts',(-0.0935296048963483,0.713513255683474,
1.129465827911));
#36698=CARTESIAN_POINT('Ctrl Pts',(-0.022059022179101,-0.563883888329778,
1.20971783562508));
#36699=CARTESIAN_POINT('Ctrl Pts',(0.0255880329657311,-1.06693159984617,
0.527617883737111));
#36700=CARTESIAN_POINT('Ctrl Pts',(0.0494115605381466,-1.11865960648645,
0.155507851120246));
#36701=CARTESIAN_POINT('Ctrl Pts',(-7.83441156053815,0.606129434160009,
-0.849820649797735));
#36702=CARTESIAN_POINT('Ctrl Pts',(-7.81058803296573,0.888813092246091,
-0.648198241866392));
#36703=CARTESIAN_POINT('Ctrl Pts',(-7.7629409778209,1.23228403552816,0.0557949640025797));
#36704=CARTESIAN_POINT('Ctrl Pts',(-7.69147039510365,0.619868497483138,
1.06785509802237));
#36705=CARTESIAN_POINT('Ctrl Pts',(-7.61999981238641,-0.560782436496941,
1.09869158672678));
#36706=CARTESIAN_POINT('Ctrl Pts',(-7.54852922966916,-1.22755265803812,
0.124845036298736));
#36707=CARTESIAN_POINT('Ctrl Pts',(-7.47705864695192,-0.770154791505453,
-0.964180713662061));
#36708=CARTESIAN_POINT('Ctrl Pts',(-7.40558806423467,0.39269579494153,-1.16968139947768));
#36709=CARTESIAN_POINT('Ctrl Pts',(-7.33411748151741,1.19584042040158,-0.304109794036846));
#36710=CARTESIAN_POINT('Ctrl Pts',(-7.26264689880018,0.903743305387708,
0.840115512674159));
#36711=CARTESIAN_POINT('Ctrl Pts',(-7.19117631608292,-0.216096822698968,
1.21482070175382));
#36712=CARTESIAN_POINT('Ctrl Pts',(-7.11970573336568,-1.13800971096765,
0.476913672937739));
#36713=CARTESIAN_POINT('Ctrl Pts',(-7.04823515064842,-1.017630262073,-0.697813105248224));
#36714=CARTESIAN_POINT('Ctrl Pts',(-6.97676456793119,0.0347913455519308,
-1.2334082688876));
#36715=CARTESIAN_POINT('Ctrl Pts',(-6.90529398521393,1.05534697353154,-0.639338172633152));
#36716=CARTESIAN_POINT('Ctrl Pts',(-6.83382340249669,1.10931796384116,0.540299980545708));
#36717=CARTESIAN_POINT('Ctrl Pts',(-6.76235281977944,0.147271992748498,
1.2250797092438));
#36718=CARTESIAN_POINT('Ctrl Pts',(-6.69088223706219,-0.949659268295102,
0.787818036098102));
#36719=CARTESIAN_POINT('Ctrl Pts',(-6.61941165434494,-1.17680416697311,
-0.371001165704848));
#36720=CARTESIAN_POINT('Ctrl Pts',(-6.5479410716277,-0.326122147885015,
-1.19002273821386));
#36721=CARTESIAN_POINT('Ctrl Pts',(-6.47647048891045,0.823252897363641,
-0.91911073289925));
#36722=CARTESIAN_POINT('Ctrl Pts',(-6.40499990619321,1.21861625625295,0.193608559273054));
#36723=CARTESIAN_POINT('Ctrl Pts',(-6.33352932347596,0.497857319454841,
1.12900306749702));
#36724=CARTESIAN_POINT('Ctrl Pts',(-6.26205874075871,-0.678885727099582,
1.03035140674798));
#36725=CARTESIAN_POINT('Ctrl Pts',(-6.19058815804147,-1.23384198279241,
-0.0119920654492216));
#36726=CARTESIAN_POINT('Ctrl Pts',(-6.11911757532421,-0.658730808215703,
-1.0433520826782));
#36727=CARTESIAN_POINT('Ctrl Pts',(-6.04764699260697,0.519707405905856,
-1.1191130687058));
#36728=CARTESIAN_POINT('Ctrl Pts',(-5.97617640988972,1.22214916322125,-0.169886051378017));
#36729=CARTESIAN_POINT('Ctrl Pts',(-5.90470582717248,0.805232864315218,
0.934938437347007));
#36730=CARTESIAN_POINT('Ctrl Pts',(-5.83323524445522,-0.349190705207747,
1.1834592088918));
#36731=CARTESIAN_POINT('Ctrl Pts',(-5.76176466173799,-1.18379289717498,
0.348057788582894));
#36732=CARTESIAN_POINT('Ctrl Pts',(-5.69029407902073,-0.934167274631489,
-0.806127378634508));
#36733=CARTESIAN_POINT('Ctrl Pts',(-5.61882349630348,0.171055762759161,
-1.22198599568372));
#36734=CARTESIAN_POINT('Ctrl Pts',(-5.54735291358624,1.11960999748104,-0.518636000621784));
#36735=CARTESIAN_POINT('Ctrl Pts',(-5.47588233086899,1.04272109636754,0.659729158662641));
#36736=CARTESIAN_POINT('Ctrl Pts',(-5.40441174815175,0.0108110778445307,
1.23385289568953));
#36737=CARTESIAN_POINT('Ctrl Pts',(-5.3329411654345,-1.03100073290279,0.677899208110117));
#36738=CARTESIAN_POINT('Ctrl Pts',(-5.26147058271725,-1.12852602694064,
-0.498937725693461));
#36739=CARTESIAN_POINT('Ctrl Pts',(-5.19,-0.192442054770818,-1.21880101048488));
#36740=CARTESIAN_POINT('Ctrl Pts',(-5.11852941728275,0.919898278591243,
-0.822372789340543));
#36741=CARTESIAN_POINT('Ctrl Pts',(-5.04705883456551,1.18971007293662,0.327261042527343));
#36742=CARTESIAN_POINT('Ctrl Pts',(-4.97558825184826,0.369874551994385,
1.17715872480732));
#36743=CARTESIAN_POINT('Ctrl Pts',(-4.90411766913101,-0.788726540276575,
0.948904785669409));
#36744=CARTESIAN_POINT('Ctrl Pts',(-4.83264708641377,-1.22493839111908,
-0.148444553842822));
#36745=CARTESIAN_POINT('Ctrl Pts',(-4.76117650369652,-0.539237551098138,
-1.10983454221279));
#36746=CARTESIAN_POINT('Ctrl Pts',(-4.68970592097927,0.640347272275161,
-1.05473466734186));
#36747=CARTESIAN_POINT('Ctrl Pts',(-4.61823533826202,1.23344241050686,-0.0336105276069657));
#36748=CARTESIAN_POINT('Ctrl Pts',(-4.54676475554478,0.696836084706056,
1.01829726438527));
#36749=CARTESIAN_POINT('Ctrl Pts',(-4.47529417282753,-0.47799764302072,
1.13755355956088));
#36750=CARTESIAN_POINT('Ctrl Pts',(-4.40382359011028,-1.21503660017309,
0.214932333172088));
#36751=CARTESIAN_POINT('Ctrl Pts',(-4.33235300739304,-0.839231849037084,
-0.904543946508284));
#36752=CARTESIAN_POINT('Ctrl Pts',(-4.26088242467578,0.305219610241788,
-1.19555461486577));
#36753=CARTESIAN_POINT('Ctrl Pts',(-4.18941184195855,1.17012251694585,-0.391564991973613));
#36754=CARTESIAN_POINT('Ctrl Pts',(-4.11794125924129,0.963318216867623,
0.771056327808787));
#36755=CARTESIAN_POINT('Ctrl Pts',(-4.04647067652406,-0.125782646596431,
1.22747243285468));
#36756=CARTESIAN_POINT('Ctrl Pts',(-3.97500009380679,-1.09968004470252,
0.559654935550513));
#36757=CARTESIAN_POINT('Ctrl Pts',(-3.90352951108956,-1.06638801435588,
-0.620746687821297));
#36758=CARTESIAN_POINT('Ctrl Pts',(-3.8320589283723,-0.0563984983524121,
-1.23261066723705));
#36759=CARTESIAN_POINT('Ctrl Pts',(-3.76058834565506,1.00524601638892,-0.715534970589979));
#36760=CARTESIAN_POINT('Ctrl Pts',(-3.68911776293781,1.14619258305115,0.456894309618231));
#36761=CARTESIAN_POINT('Ctrl Pts',(-3.61764718022056,0.237349205646206,
1.21085721791717));
#36762=CARTESIAN_POINT('Ctrl Pts',(-3.54617659750332,-0.888880685163351,
0.855804285538767));
#36763=CARTESIAN_POINT('Ctrl Pts',(-3.47470601478607,-1.20099083854098,
-0.283073936178549));
#36764=CARTESIAN_POINT('Ctrl Pts',(-3.40323543206882,-0.41312170060186,
-1.16268667666522));
#36765=CARTESIAN_POINT('Ctrl Pts',(-3.33176484935158,0.753122776159715,
-0.977402645603371));
#36766=CARTESIAN_POINT('Ctrl Pts',(-3.26029426663433,1.22958725543099,0.103077780751569));
#36767=CARTESIAN_POINT('Ctrl Pts',(-3.18882368391708,0.579881180825104,
1.08914997301927));
#36768=CARTESIAN_POINT('Ctrl Pts',(-3.11735310119984,-0.60093409949864,
1.07767715743758));
#36769=CARTESIAN_POINT('Ctrl Pts',(-3.04588251848258,-1.23135794994468,
0.0791672072957683));
#36770=CARTESIAN_POINT('Ctrl Pts',(-2.97441193576534,-0.733989479524334,
-0.991851446311691));
#36771=CARTESIAN_POINT('Ctrl Pts',(-2.90294135304809,0.435634932916331,
-1.15444014692229));
#36772=CARTESIAN_POINT('Ctrl Pts',(-2.83147077033084,1.20626429110306,-0.259685016149587));
#36773=CARTESIAN_POINT('Ctrl Pts',(-2.7600001876136,0.872084438854716,0.872913844036455));
#36774=CARTESIAN_POINT('Ctrl Pts',(-2.68852960489635,-0.260831583758772,
1.20601688732655));
#36775=CARTESIAN_POINT('Ctrl Pts',(-2.61705902217911,-1.1548537435309,0.434537315607708));
#36776=CARTESIAN_POINT('Ctrl Pts',(-2.54558843946186,-0.991153261616114,
-0.734932010182651));
#36777=CARTESIAN_POINT('Ctrl Pts',(-2.47411785674461,0.08033771071057,-1.23128213657162));
#36778=CARTESIAN_POINT('Ctrl Pts',(-2.40264727402736,1.07824792350225,-0.599909379044461));
#36779=CARTESIAN_POINT('Ctrl Pts',(-2.33117669131011,1.08859824100219,0.580916273909186));
#36780=CARTESIAN_POINT('Ctrl Pts',(-2.25970610859287,0.101908878229005,
1.22968468646956));
#36781=CARTESIAN_POINT('Ctrl Pts',(-2.18823552587562,-0.978118128803457,
0.752193308735518));
#36782=CARTESIAN_POINT('Ctrl Pts',(-2.11676494315837,-1.16229343438632,
-0.414226773643003));
#36783=CARTESIAN_POINT('Ctrl Pts',(-2.04529436044113,-0.281932136312642,
-1.20125938834656));
#36784=CARTESIAN_POINT('Ctrl Pts',(-1.97382377772388,0.856648876268221,
-0.888066748833407));
#36785=CARTESIAN_POINT('Ctrl Pts',(-1.90235319500663,1.21063104471409,0.238500149452261));
#36786=CARTESIAN_POINT('Ctrl Pts',(-1.83088261228938,0.455804522831336,
1.14662639267054));
#36787=CARTESIAN_POINT('Ctrl Pts',(-1.75941202957214,-0.71649024243284,
1.00456536876091));
#36788=CARTESIAN_POINT('Ctrl Pts',(-1.68794144685489,-1.23255649769735,
-0.0575702031048387));
#36789=CARTESIAN_POINT('Ctrl Pts',(-1.61647086413764,-0.61973268944933,
-1.06697761914173));
#36790=CARTESIAN_POINT('Ctrl Pts',(-1.54500028142039,0.560700046760855,
-1.09914753591009));
#36791=CARTESIAN_POINT('Ctrl Pts',(-1.47352969870315,1.22759145015792,-0.124615742770522));
#36792=CARTESIAN_POINT('Ctrl Pts',(-1.4020591159859,0.7701402375014,0.964050751534233));
#36793=CARTESIAN_POINT('Ctrl Pts',(-1.33058853326865,-0.392677136576001,
1.16974976838562));
#36794=CARTESIAN_POINT('Ctrl Pts',(-1.2591179505514,-1.19584423180567,0.304082958426382));
#36795=CARTESIAN_POINT('Ctrl Pts',(-1.18764736783416,-0.903745732672346,
-0.840091318538458));
#36796=CARTESIAN_POINT('Ctrl Pts',(-1.11617678511691,0.216087213885371,
-1.21483176956931));
#36797=CARTESIAN_POINT('Ctrl Pts',(-1.04470620239966,1.13800752174592,-0.476915992927436));
#36798=CARTESIAN_POINT('Ctrl Pts',(-0.973235619682416,1.01763421978166,
0.697803646148666));
#36799=CARTESIAN_POINT('Ctrl Pts',(-0.90176503696517,-0.0347827174524657,
1.23341014121216));
#36800=CARTESIAN_POINT('Ctrl Pts',(-0.830294454247921,-1.05534350947085,
0.639343890676872));
#36801=CARTESIAN_POINT('Ctrl Pts',(-0.758823871530676,-1.10932029956929,
-0.540291466200541));
#36802=CARTESIAN_POINT('Ctrl Pts',(-0.687353288813426,-0.147282209270845,
-1.22508058142116));
#36803=CARTESIAN_POINT('Ctrl Pts',(-0.615882706096181,0.949658225728546,
-0.787821050745502));
#36804=CARTESIAN_POINT('Ctrl Pts',(-0.544412123378933,1.17679880655445,
0.370987524159838));
#36805=CARTESIAN_POINT('Ctrl Pts',(-0.472941540661687,0.326144715892325,
1.19003178989654));
#36806=CARTESIAN_POINT('Ctrl Pts',(-0.401470957944438,-0.823274917779561,
0.919094928530463));
#36807=CARTESIAN_POINT('Ctrl Pts',(-0.330000375227192,-1.21856429838018,
-0.193560363613141));
#36808=CARTESIAN_POINT('Ctrl Pts',(-0.258529792509943,-0.497965769938443,
-1.12907614599118));
#36809=CARTESIAN_POINT('Ctrl Pts',(-0.187059209792698,0.679070994832269,
-1.03021084993432));
#36810=CARTESIAN_POINT('Ctrl Pts',(-0.11558862707545,1.23347601053973,0.0117079140166205));
#36811=CARTESIAN_POINT('Ctrl Pts',(-0.0441180443582029,0.659445660790309,
1.04387876930667));
#36812=CARTESIAN_POINT('Ctrl Pts',(0.0273525383590445,-0.521154695286574,
1.11804955427136));
#36813=CARTESIAN_POINT('Ctrl Pts',(0.0749995935038766,-0.986083171229488,
0.487636804522315));
#36814=CARTESIAN_POINT('Ctrl Pts',(0.098823121076292,-1.03389140639336,
0.143723997869997));
#36815=CARTESIAN_POINT('Ctrl Pts',(-7.785,0.556433207999845,-0.780144311992981));
#36816=CARTESIAN_POINT('Ctrl Pts',(-7.76117647242759,0.815939785066093,
-0.595052816798781));
#36817=CARTESIAN_POINT('Ctrl Pts',(-7.71352941728275,1.13124973052358,0.0512203649262202));
#36818=CARTESIAN_POINT('Ctrl Pts',(-7.64205883456552,0.569045812913815,
0.980302233127841));
#36819=CARTESIAN_POINT('Ctrl Pts',(-7.57058825184826,-0.514804186274824,
1.00861045471588));
#36820=CARTESIAN_POINT('Ctrl Pts',(-7.49911766913102,-1.12690627612808,
0.114609058949306));
#36821=CARTESIAN_POINT('Ctrl Pts',(-7.42764708641376,-0.70701021455541,
-0.88512805575604));
#36822=CARTESIAN_POINT('Ctrl Pts',(-7.35617650369652,0.360498878016349,
-1.07377985091759));
#36823=CARTESIAN_POINT('Ctrl Pts',(-7.28470592097927,1.09779410779162,-0.279175995659392));
#36824=CARTESIAN_POINT('Ctrl Pts',(-7.21323533826203,0.829645878065874,
0.771234893840035));
#36825=CARTESIAN_POINT('Ctrl Pts',(-7.14176475554478,-0.198379160483441,
1.11521820608871));
#36826=CARTESIAN_POINT('Ctrl Pts',(-7.07029417282753,-1.04470490710658,
0.43781177751165));
#36827=CARTESIAN_POINT('Ctrl Pts',(-6.99882359011028,-0.93419530445292,
-0.640599784228763));
#36828=CARTESIAN_POINT('Ctrl Pts',(-6.92735300739304,0.0319388218506953,
-1.1322817885948));
#36829=CARTESIAN_POINT('Ctrl Pts',(-6.85588242467578,0.968819643033635,
-0.586919179874541));
#36830=CARTESIAN_POINT('Ctrl Pts',(-6.78441184195855,1.0183655808885,0.496001075865819));
#36831=CARTESIAN_POINT('Ctrl Pts',(-6.71294125924129,0.135197241307266,
1.12463608307476));
#36832=CARTESIAN_POINT('Ctrl Pts',(-6.64147067652406,-0.871797215881005,
0.723225259228162));
#36833=CARTESIAN_POINT('Ctrl Pts',(-6.57000009380679,-1.0803186265387,-0.340582979757321));
#36834=CARTESIAN_POINT('Ctrl Pts',(-6.49852951108958,-0.299383568459973,
-1.09245341423609));
#36835=CARTESIAN_POINT('Ctrl Pts',(-6.42705892837228,0.755754835285377,
-0.843753338464662));
#36836=CARTESIAN_POINT('Ctrl Pts',(-6.35558834565508,1.11870256511677,0.177734697675315));
#36837=CARTESIAN_POINT('Ctrl Pts',(-6.28411776293779,0.457038265720188,
1.03643671348781));
#36838=CARTESIAN_POINT('Ctrl Pts',(-6.21264718022058,-0.623224251630068,
0.945873449321006));
#36839=CARTESIAN_POINT('Ctrl Pts',(-6.14117659750331,-1.13267994252993,
-0.0110088424557517));
#36840=CARTESIAN_POINT('Ctrl Pts',(-6.06970601478608,-0.604721823700482,
-0.957808206827138));
#36841=CARTESIAN_POINT('Ctrl Pts',(-5.99823543206882,0.47709687534022,-1.02735759037585));
#36842=CARTESIAN_POINT('Ctrl Pts',(-5.92676484935158,1.12194581094373,-0.155957185437944));
#36843=CARTESIAN_POINT('Ctrl Pts',(-5.85529426663432,0.739212255050342,
0.858283337941351));
#36844=CARTESIAN_POINT('Ctrl Pts',(-5.78382368391709,-0.320560747180587,
1.08642802515142));
#36845=CARTESIAN_POINT('Ctrl Pts',(-5.71235310119983,-1.08673435451183,
0.319520717780182));
#36846=CARTESIAN_POINT('Ctrl Pts',(-5.64088251848259,-0.857575402441912,
-0.740033428621935));
#36847=CARTESIAN_POINT('Ctrl Pts',(-5.56941193576534,0.157030992812372,
-1.1217960214248));
#36848=CARTESIAN_POINT('Ctrl Pts',(-5.49794135304809,1.02781377622821,-0.476113313998863));
#36849=CARTESIAN_POINT('Ctrl Pts',(-5.42647077033084,0.957228954744552,
0.605638319931491));
#36850=CARTESIAN_POINT('Ctrl Pts',(-5.3550001876136,0.00992468338927851,
1.13268996068449));
#36851=CARTESIAN_POINT('Ctrl Pts',(-5.28352960489635,-0.946469537573792,
0.6223186168017));
#36852=CARTESIAN_POINT('Ctrl Pts',(-5.21205902217911,-1.03599878522995,
-0.458030090032672));
#36853=CARTESIAN_POINT('Ctrl Pts',(-5.14058843946185,-0.176663834249519,
-1.11887217144864));
#36854=CARTESIAN_POINT('Ctrl Pts',(-5.06911785674461,0.844476313709149,
-0.754946886845504));
#36855=CARTESIAN_POINT('Ctrl Pts',(-4.99764727402736,1.09216638421668,0.30042908574342));
#36856=CARTESIAN_POINT('Ctrl Pts',(-4.92617669131012,0.339548736498745,
1.08064411436687));
#36857=CARTESIAN_POINT('Ctrl Pts',(-4.85470610859287,-0.72405927563791,
0.871104592879805));
#36858=CARTESIAN_POINT('Ctrl Pts',(-4.78323552587562,-1.12450635154704,
-0.136273664748425));
#36859=CARTESIAN_POINT('Ctrl Pts',(-4.71176494315838,-0.495025754436958,
-1.01883980527742));
#36860=CARTESIAN_POINT('Ctrl Pts',(-4.64029436044113,0.587845543979899,
-0.968257539498959));
#36861=CARTESIAN_POINT('Ctrl Pts',(-4.56882377772388,1.13231313096107,-0.0308548185336372));
#36862=CARTESIAN_POINT('Ctrl Pts',(-4.49735319500663,0.639702869075108,
0.934807619604525));
#36863=CARTESIAN_POINT('Ctrl Pts',(-4.42588261228939,-0.438806873470812,
1.0442861553082));
#36864=CARTESIAN_POINT('Ctrl Pts',(-4.35441202957213,-1.11541640311276,
0.197310146826257));
#36865=CARTESIAN_POINT('Ctrl Pts',(-4.2829414468549,-0.770423681309061,
-0.830380875051803));
#36866=CARTESIAN_POINT('Ctrl Pts',(-4.21147086413764,0.280194818630884,
-1.09753173529789));
#36867=CARTESIAN_POINT('Ctrl Pts',(-4.1400002814204,1.07418480140191,-0.359460788975286));
#36868=CARTESIAN_POINT('Ctrl Pts',(-4.06852969870314,0.884336274609667,
0.707837834382355));
#36869=CARTESIAN_POINT('Ctrl Pts',(-3.99705911598591,-0.115469795083229,
1.12683262856426));
#36870=CARTESIAN_POINT('Ctrl Pts',(-3.92558853326865,-1.00951786955407,
0.513769128524286));
#36871=CARTESIAN_POINT('Ctrl Pts',(-3.85411795055141,-0.978955434861744,
-0.569852000898709));
#36872=CARTESIAN_POINT('Ctrl Pts',(-3.78264736783416,-0.0517744158194337,
-1.13154958187441));
#36873=CARTESIAN_POINT('Ctrl Pts',(-3.71117678511691,0.922826436408769,
-0.65686864336692));
#36874=CARTESIAN_POINT('Ctrl Pts',(-3.63970620239967,1.05221686991099,0.419433791018696));
#36875=CARTESIAN_POINT('Ctrl Pts',(-3.56823561968242,0.217889071988309,
1.11157968615915));
#36876=CARTESIAN_POINT('Ctrl Pts',(-3.49676503696517,-0.816001836076439,
0.785637352659282));
#36877=CARTESIAN_POINT('Ctrl Pts',(-3.42529445424792,-1.1025222459191,-0.25986485646793));
#36878=CARTESIAN_POINT('Ctrl Pts',(-3.35382387153068,-0.379250074662353,
-1.06735862166481));
#36879=CARTESIAN_POINT('Ctrl Pts',(-3.28235328881343,0.69137464498329,-0.897265928611934));
#36880=CARTESIAN_POINT('Ctrl Pts',(-3.21088270609618,1.12877405797548,0.0946264889719359));
#36881=CARTESIAN_POINT('Ctrl Pts',(-3.13941212337894,0.532337034832168,
0.999851152782103));
#36882=CARTESIAN_POINT('Ctrl Pts',(-3.06794154066169,-0.551663836031854,
0.989318987176647));
#36883=CARTESIAN_POINT('Ctrl Pts',(-2.99647095794444,-1.13039957419878,
0.0726763305679285));
#36884=CARTESIAN_POINT('Ctrl Pts',(-2.92500037522719,-0.673810077043764,
-0.910530079924814));
#36885=CARTESIAN_POINT('Ctrl Pts',(-2.85352979250995,0.399917459173323,
-1.05978822045819));
#36886=CARTESIAN_POINT('Ctrl Pts',(-2.78205920979269,1.10736333094316,-0.238393581406989));
#36887=CARTESIAN_POINT('Ctrl Pts',(-2.71058862707545,0.800582704964894,
0.801344107662086));
#36888=CARTESIAN_POINT('Ctrl Pts',(-2.6391180443582,-0.239446142554869,
1.10713621166916));
#36889=CARTESIAN_POINT('Ctrl Pts',(-2.56764746164096,-1.06016790650342,
0.398909834917203));
#36890=CARTESIAN_POINT('Ctrl Pts',(-2.49617687892371,-0.909889139016734,
-0.674675330120583));
#36891=CARTESIAN_POINT('Ctrl Pts',(-2.42470629620646,0.0737508650376029,
-1.13032997672338));
#36892=CARTESIAN_POINT('Ctrl Pts',(-2.35323571348922,0.989842956438803,
-0.550723131856308));
#36893=CARTESIAN_POINT('Ctrl Pts',(-2.28176513077197,0.999344656976215,
0.533287261191272));
#36894=CARTESIAN_POINT('Ctrl Pts',(-2.21029454805472,0.0935534241382057,
1.12886350069563));
#36895=CARTESIAN_POINT('Ctrl Pts',(-2.13882396533747,-0.897922749729446,
0.690521384093054));
#36896=CARTESIAN_POINT('Ctrl Pts',(-2.06735338262023,-1.06699762110876,
-0.380264543359496));
#36897=CARTESIAN_POINT('Ctrl Pts',(-1.99588279990298,-0.258816672158623,
-1.10276877747064));
#36898=CARTESIAN_POINT('Ctrl Pts',(-1.92441221718573,0.786412695849304,
-0.815254633948207));
#36899=CARTESIAN_POINT('Ctrl Pts',(-1.85294163446849,1.11137205677529,0.218945650531032));
#36900=CARTESIAN_POINT('Ctrl Pts',(-1.78147105175124,0.418433355264041,
1.05261511171313));
#36901=CARTESIAN_POINT('Ctrl Pts',(-1.71000046903399,-0.657745592985418,
0.922201594713525));
#36902=CARTESIAN_POINT('Ctrl Pts',(-1.63852988631674,-1.13149985366612,
-0.0528500531297068));
#36903=CARTESIAN_POINT('Ctrl Pts',(-1.5670593035995,-0.568921139707624,
-0.979496698268463));
#36904=CARTESIAN_POINT('Ctrl Pts',(-1.49558872088225,0.514728551628869,
-1.00902902087099));
#36905=CARTESIAN_POINT('Ctrl Pts',(-1.424118138165,1.12694188770285,-0.114398565074092));
#36906=CARTESIAN_POINT('Ctrl Pts',(-1.35264755544776,0.706996853826318,
0.885008749153142));
#36907=CARTESIAN_POINT('Ctrl Pts',(-1.28117697273051,-0.360481749440169,
1.07384261429556));
#36908=CARTESIAN_POINT('Ctrl Pts',(-1.20970639001326,-1.09779760670074,
0.279151360286191));
#36909=CARTESIAN_POINT('Ctrl Pts',(-1.13823580729601,-0.82964810633875,
-0.771212683368502));
#36910=CARTESIAN_POINT('Ctrl Pts',(-1.06676522457877,0.1983703394913,-1.11522836645996));
#36911=CARTESIAN_POINT('Ctrl Pts',(-0.995294641861518,1.04470289737796,
-0.437813907286639));
#36912=CARTESIAN_POINT('Ctrl Pts',(-0.923824059144271,0.934198937671177,
0.640591100675686));
#36913=CARTESIAN_POINT('Ctrl Pts',(-0.852353476427024,-0.0319309011644629,
1.13228350740848));
#36914=CARTESIAN_POINT('Ctrl Pts',(-0.780882893709776,-0.968816462989413,
0.586924429098932));
#36915=CARTESIAN_POINT('Ctrl Pts',(-0.709412310992529,-1.01836772511154,
-0.49599325960723));
#36916=CARTESIAN_POINT('Ctrl Pts',(-0.637941728275282,-0.135206620182443,
-1.12463688374277));
#36917=CARTESIAN_POINT('Ctrl Pts',(-0.566471145558034,0.87179625879392,
-0.723228026706244));
#36918=CARTESIAN_POINT('Ctrl Pts',(-0.495000562840788,1.08031370561788,
0.340570456675246));
#36919=CARTESIAN_POINT('Ctrl Pts',(-0.42352998012354,0.299404286128507,
1.09246172377618));
#36920=CARTESIAN_POINT('Ctrl Pts',(-0.352059397406293,-0.755775050259243,
0.843738829887568));
#36921=CARTESIAN_POINT('Ctrl Pts',(-0.280588814689047,-1.11865486724203,
-0.177690453551626));
#36922=CARTESIAN_POINT('Ctrl Pts',(-0.209118231971798,-0.457137824406994,
-1.03650380031556));
#36923=CARTESIAN_POINT('Ctrl Pts',(-0.137647649254552,0.62339432936104,
-0.945744416684868));
#36924=CARTESIAN_POINT('Ctrl Pts',(-0.0661770665373043,1.13234397614533,
0.0107479884462148));
#36925=CARTESIAN_POINT('Ctrl Pts',(0.00529351617994261,0.605378065897145,
0.958291710702337));
#36926=CARTESIAN_POINT('Ctrl Pts',(0.07676409889719,-0.478425502243371,
1.02638127291764));
#36927=CARTESIAN_POINT('Ctrl Pts',(0.124411154042022,-0.905234742612801,
0.447655725307518));
#36928=CARTESIAN_POINT('Ctrl Pts',(0.148234681614438,-0.949123206300278,
0.131940144619747));
#36929=CARTESIAN_POINT('Ctrl Pts',(-1.11022302462516E-16,0.570663374910274,
0.771750967939225));
#36930=CARTESIAN_POINT('Ctrl Pts',(-1.6227853268113E-16,0.553554149972714,
0.78839235193671));
#36931=CARTESIAN_POINT('Ctrl Pts',(-1.23639223896832E-15,0.535816051891995,
0.804318657007652));
#36932=CARTESIAN_POINT('Ctrl Pts',(-5.55111512312578E-16,0.517476131545855,
0.819482603444016));
#36933=CARTESIAN_POINT('Ctrl Pts',(6.73446525316235E-16,0.484403631959195,
0.846827848286062));
#36934=CARTESIAN_POINT('Ctrl Pts',(1.46277561945344E-15,0.449377049094155,
0.871696546385583));
#36935=CARTESIAN_POINT('Ctrl Pts',(1.88737914186277E-15,0.412720708654321,
0.894110857505424));
#36936=CARTESIAN_POINT('Ctrl Pts',(2.02722893480718E-15,0.400647371175813,
0.901493360484473));
#36937=CARTESIAN_POINT('Ctrl Pts',(1.96982266612964E-15,0.388396839386775,
0.908609315816784));
#36938=CARTESIAN_POINT('Ctrl Pts',(1.85962356624714E-15,0.375979633652141,
0.915458615713178));
#36939=CARTESIAN_POINT('Ctrl Pts',(1.76000123446738E-15,0.364754215379286,
0.921650528600536));
#36940=CARTESIAN_POINT('Ctrl Pts',(2.82869925563963E-15,0.353389819517391,
0.9276256539064));
#36941=CARTESIAN_POINT('Ctrl Pts',(2.72004641033163E-15,0.341916629859017,
0.933372903137718));
#36942=CARTESIAN_POINT('Ctrl Pts',(2.35276881084968E-15,0.303133977235575,
0.952800244366746));
#36943=CARTESIAN_POINT('Ctrl Pts',(1.1688040584756E-15,0.263061982855837,
0.969655391781731));
#36944=CARTESIAN_POINT('Ctrl Pts',(2.08166817117217E-15,0.222016046761304,
0.983957630079311));
#36945=CARTESIAN_POINT('Ctrl Pts',(2.69006659399074E-15,0.194660077306816,
0.993489672255138));
#36946=CARTESIAN_POINT('Ctrl Pts',(1.53826374099029E-15,0.166870521404496,
1.00188706363919));
#36947=CARTESIAN_POINT('Ctrl Pts',(1.38777878078145E-15,0.138732201281755,
1.0091461379835));
#36948=CARTESIAN_POINT('Ctrl Pts',(1.33800608025447E-15,0.129425489309623,
1.01154706717231));
#36949=CARTESIAN_POINT('Ctrl Pts',(2.68620275761292E-15,0.120080580177726,
1.01382340557925));
#36950=CARTESIAN_POINT('Ctrl Pts',(2.692290834716E-15,0.110700425114071,
1.01597482323229));
#36951=CARTESIAN_POINT('Ctrl Pts',(2.6983819628624E-15,0.101315569180366,
1.01812731906951));
#36952=CARTESIAN_POINT('Ctrl Pts',(3.01944477006372E-15,0.0919037451979173,
1.02015282977562));
#36953=CARTESIAN_POINT('Ctrl Pts',(2.95596880306448E-15,0.08247156602505,
1.02205097598145));
#36954=CARTESIAN_POINT('Ctrl Pts',(2.65201403921594E-15,0.037305561809622,
1.03114025195497));
#36955=CARTESIAN_POINT('Ctrl Pts',(3.06257071685217E-15,-0.00834860240433294,
1.03731815327265));
#36956=CARTESIAN_POINT('Ctrl Pts',(3.10862446895044E-15,-0.0541501896412871,
1.04060058451353));
#36957=CARTESIAN_POINT('Ctrl Pts',(3.15460360551374E-15,-0.0998775698966539,
1.04387769761306));
#36958=CARTESIAN_POINT('Ctrl Pts',(3.03885975298288E-15,-0.145753160502293,
1.0442690927114));
#36959=CARTESIAN_POINT('Ctrl Pts',(3.48332473976143E-15,-0.191464036720484,
1.0417442192531));
#36960=CARTESIAN_POINT('Ctrl Pts',(3.70609819577921E-15,-0.214375109978547,
1.04047870947608));
#36961=CARTESIAN_POINT('Ctrl Pts',(1.06235067126326E-15,-0.237245096712249,
1.03847981622708));
#36962=CARTESIAN_POINT('Ctrl Pts',(9.0205620750794E-16,-0.260035528443775,
1.03573883777575));
#36963=CARTESIAN_POINT('Ctrl Pts',(8.33206419365417E-16,-0.269824490330739,
1.03456153082917));
#36964=CARTESIAN_POINT('Ctrl Pts',(8.13320907073322E-16,-0.279598777118199,
1.03324727556146));
#36965=CARTESIAN_POINT('Ctrl Pts',(7.63278329429795E-16,-0.289355335937033,
1.03179518646881));
#36966=CARTESIAN_POINT('Ctrl Pts',(7.23513230033157E-16,-0.297108144634533,
1.03064131970532));
#36967=CARTESIAN_POINT('Ctrl Pts',(1.46426492949664E-15,-0.304847930595704,
1.02940061940942));
#36968=CARTESIAN_POINT('Ctrl Pts',(1.4432899320127E-15,-0.312563996860672,
1.02807450029725));
#36969=CARTESIAN_POINT('Ctrl Pts',(1.31665470348709E-15,-0.359149261794851,
1.02006813953604));
#36970=CARTESIAN_POINT('Ctrl Pts',(-6.4851176683571E-16,-0.404962145828001,
1.00893866567721));
#36971=CARTESIAN_POINT('Ctrl Pts',(-6.93889390390723E-16,-0.449670173943294,
0.994677276149143));
#36972=CARTESIAN_POINT('Ctrl Pts',(-6.97600981451806E-16,-0.45332699650277,
0.993510788313419));
#36973=CARTESIAN_POINT('Ctrl Pts',(1.49899777376848E-15,-0.456976434972893,
0.992323319606125));
#36974=CARTESIAN_POINT('Ctrl Pts',(1.51267887105178E-15,-0.460618310709277,
0.991114850128469));
#36975=CARTESIAN_POINT('Ctrl Pts',(1.67393459725224E-15,-0.503544203599426,
0.976870917849112));
#36976=CARTESIAN_POINT('Ctrl Pts',(1.12125522885397E-15,-0.545419935519386,
0.959713756948874));
#36977=CARTESIAN_POINT('Ctrl Pts',(7.49400541621981E-16,-0.58610720628139,
0.939888327104482));
#36978=CARTESIAN_POINT('Ctrl Pts',(5.63148709306203E-16,-0.606486346282988,
0.929958312069705));
#36979=CARTESIAN_POINT('Ctrl Pts',(1.00622254320331E-15,-0.626567238076758,
0.919358074802143));
#36980=CARTESIAN_POINT('Ctrl Pts',(8.67361737988404E-16,-0.646331465200864,
0.908113776412865));
#36981=CARTESIAN_POINT('Ctrl Pts',(7.95690601173239E-16,-0.656532505185225,
0.902310183044663));
#36982=CARTESIAN_POINT('Ctrl Pts',(-4.50726463038882E-16,-0.666649171563993,
0.896334966382544));
#36983=CARTESIAN_POINT('Ctrl Pts',(-4.30211422042248E-16,-0.676678817816388,
0.890191433267475));
#36984=CARTESIAN_POINT('Ctrl Pts',(-4.11809703290141E-16,-0.685675277026487,
0.884680765823705));
#36985=CARTESIAN_POINT('Ctrl Pts',(-7.31588621547825E-16,-0.694602965016621,
0.879033670020616));
#36986=CARTESIAN_POINT('Ctrl Pts',(-7.49400541621981E-16,-0.703442280964398,
0.873264474759485));
#36987=CARTESIAN_POINT('Ctrl Pts',(-8.29389137610011E-16,-0.743137298077302,
0.847356553154324));
#36988=CARTESIAN_POINT('Ctrl Pts',(4.14969713553736E-16,-0.781133291997709,
0.818941549086768));
#36989=CARTESIAN_POINT('Ctrl Pts',(2.35922392732846E-16,-0.817284769458134,
0.788303358144051));
#36990=CARTESIAN_POINT('Ctrl Pts',(5.28234168389171E-17,-0.854254317339153,
0.756971856733506));
#36991=CARTESIAN_POINT('Ctrl Pts',(1.57130807400593E-15,-0.889295824999286,
0.723314911167561));
#36992=CARTESIAN_POINT('Ctrl Pts',(1.68615121864946E-15,-0.922238196069141,
0.687583577395874));
#36993=CARTESIAN_POINT('Ctrl Pts',(1.74491354597361E-15,-0.939093972682094,
0.669300759232564));
#36994=CARTESIAN_POINT('Ctrl Pts',(1.80102997402413E-15,-0.955399840771159,
0.650474053122468));
#36995=CARTESIAN_POINT('Ctrl Pts',(1.98452365651747E-15,-0.971130158053256,
0.631132646543269));
#36996=CARTESIAN_POINT('Ctrl Pts',(2.11257469800354E-15,-0.982107557838951,
0.617635248580471));
#36997=CARTESIAN_POINT('Ctrl Pts',(7.30982271506299E-16,-0.992804626999012,
0.603887133573503));
#36998=CARTESIAN_POINT('Ctrl Pts',(6.52256026967279E-16,-1.00321195432393,
0.589897488249048));
#36999=CARTESIAN_POINT('Ctrl Pts',(6.10633372201704E-16,-1.00871432008283,
0.582501146901354));
#37000=CARTESIAN_POINT('Ctrl Pts',(1.17225784430234E-15,-1.0141354010843,
0.575037484420216));
#37001=CARTESIAN_POINT('Ctrl Pts',(1.08246744900953E-15,-1.01946584908478,
0.567519513872719));
#37002=CARTESIAN_POINT('Ctrl Pts',(5.90599146279996E-16,-1.04866583648026,
0.526336362811751));
#37003=CARTESIAN_POINT('Ctrl Pts',(1.80552960326234E-15,-1.0752125083205,
0.483441946932646));
#37004=CARTESIAN_POINT('Ctrl Pts',(1.23859256184744E-15,-1.09893418145565,
0.439114326182033));
#37005=CARTESIAN_POINT('Ctrl Pts',(6.75767736099756E-16,-1.12248379203571,
0.395108230968164));
#37006=CARTESIAN_POINT('Ctrl Pts',(-8.48028993383386E-16,-1.14325009528961,
0.349688793728424));
#37007=CARTESIAN_POINT('Ctrl Pts',(-8.70831184940357E-16,-1.16103400319525,
0.303088562628634));
#37008=CARTESIAN_POINT('Ctrl Pts',(-8.92487487529703E-16,-1.17792420823819,
0.258830154268672));
#37009=CARTESIAN_POINT('Ctrl Pts',(-9.88970463367636E-16,-1.19212468288807,
0.21350576212291));
#37010=CARTESIAN_POINT('Ctrl Pts',(-9.29811783123569E-16,-1.20342780657952,
0.167291704370529));
#37011=CARTESIAN_POINT('Origin',(0.179677267864665,0.,0.));
#37012=CARTESIAN_POINT('',(-0.0506454642706703,0.,0.));
#37013=CARTESIAN_POINT('',(0.4,-0.733718498103797,8.98546010178019E-17));
#37014=CARTESIAN_POINT('',(0.179677267864665,-0.375,-4.59242549680257E-17));
#37015=CARTESIAN_POINT('Origin',(0.4,0.,0.));
#37016=CARTESIAN_POINT('Origin',(1.4,-1.38777878078145E-16,-0.866025403784439));
#37017=CARTESIAN_POINT('',(1.26393192622467,-1.59086285808736E-16,-0.866025403784439));
#37018=CARTESIAN_POINT('',(1.26393192622467,-0.75,-0.433012701892219));
#37019=CARTESIAN_POINT('Ctrl Pts',(1.26393192622467,-4.16333634234434E-16,
-0.866025403784438));
#37020=CARTESIAN_POINT('Ctrl Pts',(1.28128077719016,-0.128085793099759,
-0.792075036658926));
#37021=CARTESIAN_POINT('Ctrl Pts',(1.28802832775523,-0.255151508715124,
-0.718713611543623));
#37022=CARTESIAN_POINT('Ctrl Pts',(1.28802832775523,-0.494848491284876,
-0.580324494133036));
#37023=CARTESIAN_POINT('Ctrl Pts',(1.28128077719016,-0.621914206900241,
-0.506963069017732));
#37024=CARTESIAN_POINT('Ctrl Pts',(1.26393192622467,-0.75,-0.43301270189222));
#37025=CARTESIAN_POINT('',(0.4,-1.38777878078145E-16,-0.866025403784439));
#37026=CARTESIAN_POINT('',(1.4,-1.59086285808736E-16,-0.866025403784439));
#37027=CARTESIAN_POINT('',(0.4,-0.75,-0.433012701892219));
#37028=CARTESIAN_POINT('',(0.4,-0.75,-0.433012701892219));
#37029=CARTESIAN_POINT('',(1.4,-0.75,-0.433012701892219));
#37030=CARTESIAN_POINT('Origin',(1.4,-0.75,-0.433012701892219));
#37031=CARTESIAN_POINT('',(1.26393192622467,-0.75,0.433012701892219));
#37032=CARTESIAN_POINT('Ctrl Pts',(1.26393192622467,-0.75,-0.433012701892219));
#37033=CARTESIAN_POINT('Ctrl Pts',(1.28128077719016,-0.75,-0.285111967641195));
#37034=CARTESIAN_POINT('Ctrl Pts',(1.28802832775523,-0.75,-0.138389117410587));
#37035=CARTESIAN_POINT('Ctrl Pts',(1.28802832775523,-0.75,0.138389117410587));
#37036=CARTESIAN_POINT('Ctrl Pts',(1.28128077719016,-0.75,0.285111967641195));
#37037=CARTESIAN_POINT('Ctrl Pts',(1.26393192622467,-0.75,0.433012701892219));
#37038=CARTESIAN_POINT('',(0.4,-0.75,0.433012701892219));
#37039=CARTESIAN_POINT('',(0.4,-0.75,0.433012701892219));
#37040=CARTESIAN_POINT('',(1.4,-0.75,0.433012701892219));
#37041=CARTESIAN_POINT('Origin',(1.4,-0.75,0.433012701892219));
#37042=CARTESIAN_POINT('',(1.26393192622467,5.30287619362453E-17,0.866025403784439));
#37043=CARTESIAN_POINT('Ctrl Pts',(1.26393192622467,-0.75,0.433012701892219));
#37044=CARTESIAN_POINT('Ctrl Pts',(1.28128077719016,-0.621914206900242,
0.506963069017732));
#37045=CARTESIAN_POINT('Ctrl Pts',(1.28802832775523,-0.494848491284876,
0.580324494133036));
#37046=CARTESIAN_POINT('Ctrl Pts',(1.28802832775523,-0.255151508715124,
0.718713611543623));
#37047=CARTESIAN_POINT('Ctrl Pts',(1.28128077719016,-0.128085793099759,
0.792075036658926));
#37048=CARTESIAN_POINT('Ctrl Pts',(1.26393192622467,-2.42861286636753E-16,
0.866025403784438));
#37049=CARTESIAN_POINT('',(0.4,0.,0.866025403784439));
#37050=CARTESIAN_POINT('',(0.4,5.30287619362453E-17,0.866025403784439));
#37051=CARTESIAN_POINT('',(1.4,5.30287619362453E-17,0.866025403784439));
#37052=CARTESIAN_POINT('Origin',(1.4,0.,0.866025403784439));
#37053=CARTESIAN_POINT('',(1.26393192622467,0.75,0.433012701892219));
#37054=CARTESIAN_POINT('Ctrl Pts',(1.26393192622467,2.94902990916057E-16,
0.866025403784438));
#37055=CARTESIAN_POINT('Ctrl Pts',(1.28128077719016,0.128085793099758,0.792075036658926));
#37056=CARTESIAN_POINT('Ctrl Pts',(1.28802832775523,0.255151508715124,0.718713611543623));
#37057=CARTESIAN_POINT('Ctrl Pts',(1.28802832775523,0.494848491284876,0.580324494133036));
#37058=CARTESIAN_POINT('Ctrl Pts',(1.28128077719016,0.621914206900242,0.506963069017732));
#37059=CARTESIAN_POINT('Ctrl Pts',(1.26393192622467,0.75,0.433012701892219));
#37060=CARTESIAN_POINT('',(0.4,0.75,0.433012701892219));
#37061=CARTESIAN_POINT('',(0.4,0.75,0.433012701892219));
#37062=CARTESIAN_POINT('',(1.4,0.75,0.433012701892219));
#37063=CARTESIAN_POINT('Origin',(1.4,0.75,-0.43301270189222));
#37064=CARTESIAN_POINT('',(1.26393192622467,0.75,-0.43301270189222));
#37065=CARTESIAN_POINT('Ctrl Pts',(1.26393192622467,0.749999999999999,-0.43301270189222));
#37066=CARTESIAN_POINT('Ctrl Pts',(1.28128077719016,0.621914206900241,-0.506963069017732));
#37067=CARTESIAN_POINT('Ctrl Pts',(1.28802832775523,0.494848491284876,-0.580324494133036));
#37068=CARTESIAN_POINT('Ctrl Pts',(1.28802832775523,0.255151508715124,-0.718713611543623));
#37069=CARTESIAN_POINT('Ctrl Pts',(1.28128077719016,0.128085793099758,-0.792075036658926));
#37070=CARTESIAN_POINT('Ctrl Pts',(1.26393192622467,1.38777878078145E-16,
-0.866025403784438));
#37071=CARTESIAN_POINT('',(0.4,0.75,-0.43301270189222));
#37072=CARTESIAN_POINT('',(1.4,0.75,-0.43301270189222));
#37073=CARTESIAN_POINT('',(0.4,-1.59086285808736E-16,-0.866025403784439));
#37074=CARTESIAN_POINT('Origin',(1.4,0.75,0.433012701892219));
#37075=CARTESIAN_POINT('Ctrl Pts',(1.26393192622467,0.75,0.433012701892219));
#37076=CARTESIAN_POINT('Ctrl Pts',(1.28128077719016,0.75,0.285111967641195));
#37077=CARTESIAN_POINT('Ctrl Pts',(1.28802832775523,0.75,0.138389117410587));
#37078=CARTESIAN_POINT('Ctrl Pts',(1.28802832775523,0.75,-0.138389117410587));
#37079=CARTESIAN_POINT('Ctrl Pts',(1.28128077719016,0.75,-0.285111967641195));
#37080=CARTESIAN_POINT('Ctrl Pts',(1.26393192622467,0.75,-0.433012701892219));
#37081=CARTESIAN_POINT('',(0.4,0.75,-0.43301270189222));
#37082=CARTESIAN_POINT('Origin',(0.4,0.,0.));
#37083=CARTESIAN_POINT('Origin',(-8.,1.,0.));
#37084=CARTESIAN_POINT('',(-8.,-1.,-1.22464679914735E-16));
#37085=CARTESIAN_POINT('Origin',(-8.,0.,0.));
#37086=CARTESIAN_POINT('Origin',(-7.875,0.,0.));
#37087=CARTESIAN_POINT('',(-7.875,-1.125,-1.37772764904077E-16));
#37088=CARTESIAN_POINT('Origin',(-3.875,0.,0.));
#37089=CARTESIAN_POINT('Origin',(0.,0.,0.));
#37090=CARTESIAN_POINT('Origin',(0.,2.35,0.));
#37091=CARTESIAN_POINT('',(-8.67361737988404E-18,-2.35,-2.87791997799628E-16));
#37092=CARTESIAN_POINT('Origin',(0.,0.,0.));
#37093=CARTESIAN_POINT('Origin',(0.0749999999999999,0.,0.));
#37094=CARTESIAN_POINT('',(0.15,-2.35,-2.87791997799628E-16));
#37095=CARTESIAN_POINT('',(0.15,-2.87791997799628E-16,2.35));
#37096=CARTESIAN_POINT('Origin',(0.15,0.,0.));
#37097=CARTESIAN_POINT('',(0.0749999999999999,-2.35,-2.87791997799628E-16));
#37098=CARTESIAN_POINT('Origin',(0.15,0.,0.));
#37099=CARTESIAN_POINT('Ctrl Pts',(0.15,0.,2.35));
#37100=CARTESIAN_POINT('Ctrl Pts',(0.15,-2.35,2.35));
#37101=CARTESIAN_POINT('Ctrl Pts',(0.15,-2.35,0.));
#37102=CARTESIAN_POINT('Ctrl Pts',(0.15,-2.35,-2.35));
#37103=CARTESIAN_POINT('Ctrl Pts',(0.15,0.,-2.35));
#37104=CARTESIAN_POINT('Ctrl Pts',(0.15,2.35,-2.35));
#37105=CARTESIAN_POINT('Ctrl Pts',(0.15,2.35,0.));
#37106=CARTESIAN_POINT('Ctrl Pts',(0.15,2.35,2.35));
#37107=CARTESIAN_POINT('Ctrl Pts',(0.15,0.,2.35));
#37108=CARTESIAN_POINT('Ctrl Pts',(1.09479837717015,0.,1.81728317490632));
#37109=CARTESIAN_POINT('Ctrl Pts',(1.09479837717015,-1.81728317490632,1.81728317490632));
#37110=CARTESIAN_POINT('Ctrl Pts',(1.09479837717015,-1.81728317490632,0.));
#37111=CARTESIAN_POINT('Ctrl Pts',(1.09479837717015,-1.81728317490632,-1.81728317490632));
#37112=CARTESIAN_POINT('Ctrl Pts',(1.09479837717015,0.,-1.81728317490632));
#37113=CARTESIAN_POINT('Ctrl Pts',(1.09479837717015,1.81728317490632,-1.81728317490632));
#37114=CARTESIAN_POINT('Ctrl Pts',(1.09479837717015,1.81728317490632,0.));
#37115=CARTESIAN_POINT('Ctrl Pts',(1.09479837717015,1.81728317490632,1.81728317490632));
#37116=CARTESIAN_POINT('Ctrl Pts',(1.09479837717015,0.,1.81728317490632));
#37117=CARTESIAN_POINT('Ctrl Pts',(1.28802832775523,0.,0.75));
#37118=CARTESIAN_POINT('Ctrl Pts',(1.28802832775523,-0.75,0.75));
#37119=CARTESIAN_POINT('Ctrl Pts',(1.28802832775523,-0.75,0.));
#37120=CARTESIAN_POINT('Ctrl Pts',(1.28802832775523,-0.75,-0.75));
#37121=CARTESIAN_POINT('Ctrl Pts',(1.28802832775523,0.,-0.75));
#37122=CARTESIAN_POINT('Ctrl Pts',(1.28802832775523,0.75,-0.75));
#37123=CARTESIAN_POINT('Ctrl Pts',(1.28802832775523,0.75,0.));
#37124=CARTESIAN_POINT('Ctrl Pts',(1.28802832775523,0.75,0.75));
#37125=CARTESIAN_POINT('Ctrl Pts',(1.28802832775523,0.,0.75));
#37126=CARTESIAN_POINT('Ctrl Pts',(1.26393192622467,0.,0.86602540378444));
#37127=CARTESIAN_POINT('Ctrl Pts',(1.03252872779688,0.,1.85239340658685));
#37128=CARTESIAN_POINT('Ctrl Pts',(0.15,0.,2.35));
#37165=UNCERTAINTY_MEASURE_WITH_UNIT(LENGTH_MEASURE(0.01),#37182,
'DISTANCE_ACCURACY_VALUE',
'Maximum model space distance between geometric entities at asserted c
onnectivities');
#37166=UNCERTAINTY_MEASURE_WITH_UNIT(LENGTH_MEASURE(0.01),#37182,
'DISTANCE_ACCURACY_VALUE',
'Maximum model space distance between geometric entities at asserted c
onnectivities');
#37180=(
GEOMETRIC_REPRESENTATION_CONTEXT(3)
GLOBAL_UNCERTAINTY_ASSIGNED_CONTEXT((#37165))
GLOBAL_UNIT_ASSIGNED_CONTEXT((#37182,#37184,#37185))
REPRESENTATION_CONTEXT('','3D')
);
#37181=(
GEOMETRIC_REPRESENTATION_CONTEXT(3)
GLOBAL_UNCERTAINTY_ASSIGNED_CONTEXT((#37166))
GLOBAL_UNIT_ASSIGNED_CONTEXT((#37182,#37184,#37185))
REPRESENTATION_CONTEXT('','3D')
);
#37182=(
LENGTH_UNIT()
NAMED_UNIT(*)
SI_UNIT(.MILLI.,.METRE.)
);
#37184=(
NAMED_UNIT(*)
PLANE_ANGLE_UNIT()
SI_UNIT($,.RADIAN.)
);
#37185=(
NAMED_UNIT(*)
SI_UNIT($,.STERADIAN.)
SOLID_ANGLE_UNIT()
);
#37199=SHAPE_DEFINITION_REPRESENTATION(#37213,#37250);
#37213=PRODUCT_DEFINITION_SHAPE('',$,#37265);
#37250=SHAPE_REPRESENTATION('',(#16039),#37180);
#37251=PRODUCT_DEFINITION_CONTEXT('part definition',#37295,'design');
#37265=PRODUCT_DEFINITION('2026-10-20-13-24-05-459',
'13_ISO_7380_M2.5x8',#37279,#37251);
#37279=PRODUCT_DEFINITION_FORMATION('',$,#37310);
#37295=APPLICATION_CONTEXT(
'Core Data for Automotive Mechanical Design Process');
#37296=PRODUCT_CONTEXT('part definition',#37295,'mechanical');
#37310=PRODUCT('2026-10-20-13-24-05-459','13_ISO_7380_M2.5x8',$,(#37296));
#37374=COLOUR_RGB('Black',0.12,0.14,0.17);
#37375=FILL_AREA_STYLE_COLOUR('',#37374);
#37376=FILL_AREA_STYLE('',(#37375));
#37377=SURFACE_STYLE_FILL_AREA(#37376);
#37378=SURFACE_SIDE_STYLE('',(#37377));
#37379=SURFACE_STYLE_USAGE(.BOTH.,#37378);
#37380=PRESENTATION_STYLE_ASSIGNMENT((#37379));
ENDSEC;
END-ISO-10303-21;
